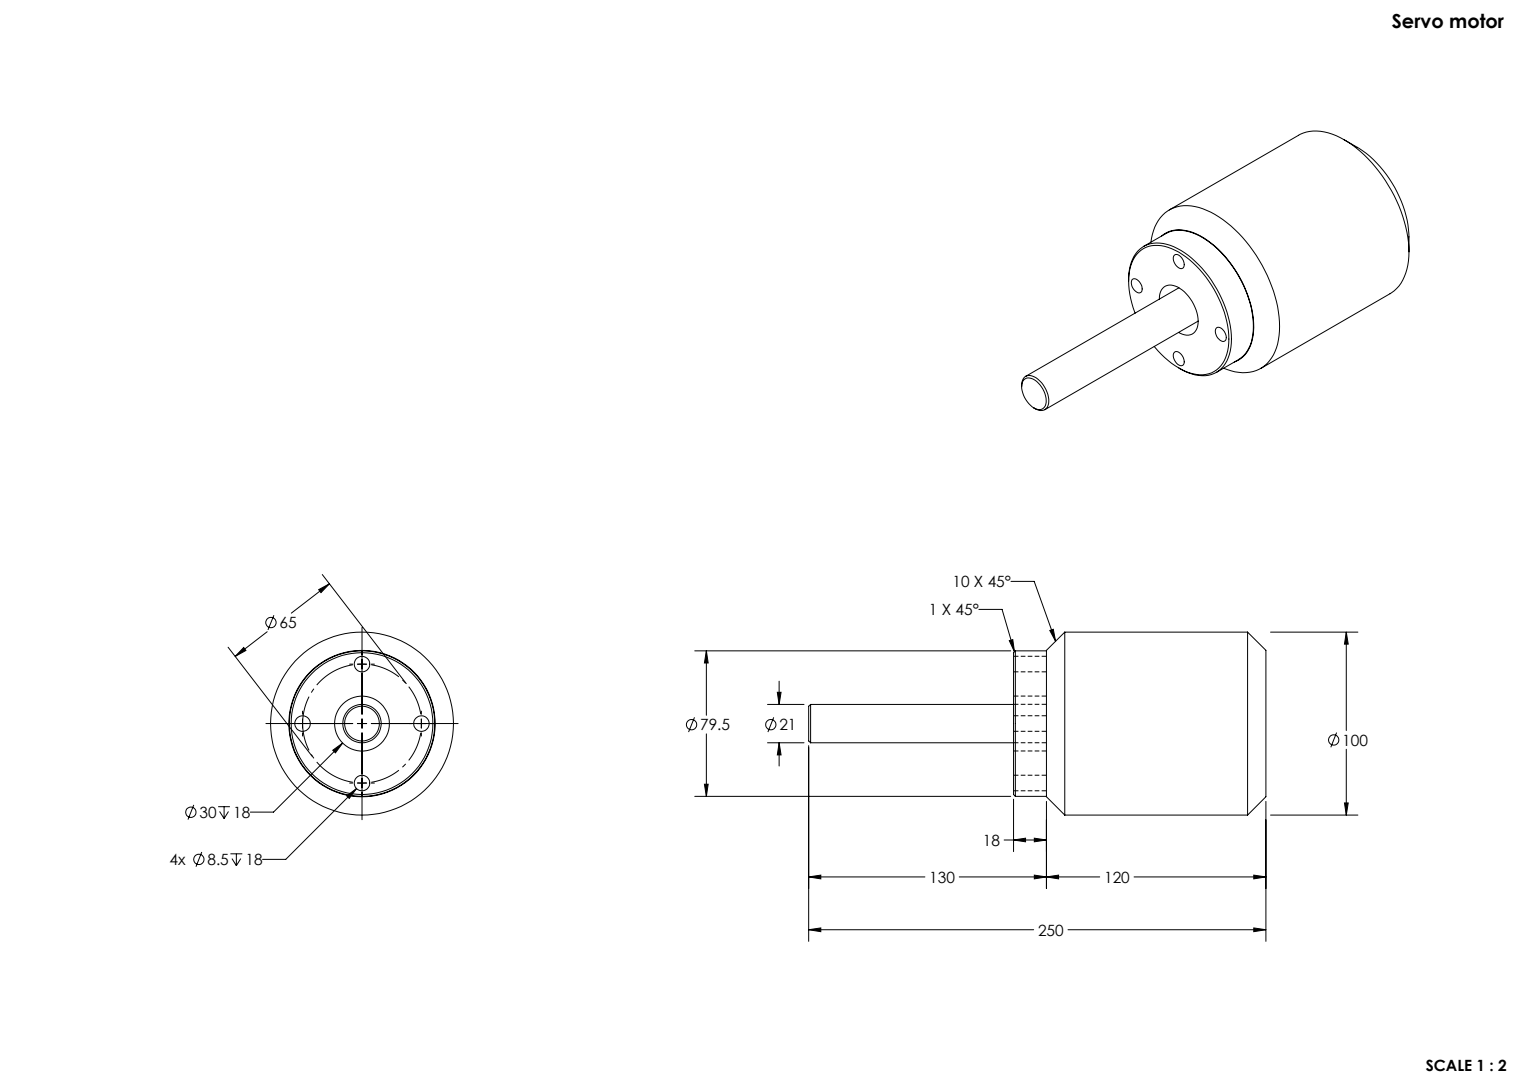
ISO-10303-21;
HEADER;
FILE_DESCRIPTION (('STEP AP214'),
    '1' );
FILE_NAME ('Servo motor.step',
    '2026-10-24T15:53:57',
    ( '' ),
    ( '' ),
    'SwSTEP 2.0',
    'SolidWorks 2025',
    '' );
FILE_SCHEMA (( 'AUTOMOTIVE_DESIGN' ));
ENDSEC;

DATA;
#2=DIRECTION ( 'NONE',  ( -3.851859888774471706E-33, -1.232595164407830946E-32, -1.000000000000000000 ) ) ;
#12=CONICAL_SURFACE ( 'NONE', #4068, 9.499999999999998224, 0.7853981633974257415 ) ;
#15=CIRCLE ( 'NONE', #7701, 10.50000000000002132 ) ;
#24=CARTESIAN_POINT ( 'NONE',  ( 28.24999999999996092, 1.387778780781445676E-14, 18.00000000000000355 ) ) ;
#39=EDGE_CURVE ( 'NONE', #7000, #2703, #3383, .T. ) ;
#42=ORIENTED_EDGE ( 'NONE', *, *, #2072, .T. ) ;
#43=CARTESIAN_POINT ( 'NONE',  ( 15.00000000000000000, 1.836970198721029589E-15, -4.814824860968080875E-32 ) ) ;
#49=DIRECTION ( 'NONE',  ( 3.851859888774471706E-33, -7.598173571352223877E-18, 1.000000000000000000 ) ) ;
#50=ORIENTED_EDGE ( 'NONE', *, *, #3725, .T. ) ;
#58=DIRECTION ( 'NONE',  ( -3.851859888774471706E-33, 7.598173571352223877E-18, -1.000000000000000000 ) ) ;
#68=ORIENTED_EDGE ( 'NONE', *, *, #5960, .T. ) ;
#70=CIRCLE ( 'NONE', #2861, 15.00000000000002487 ) ;
#72=DIRECTION ( 'NONE',  ( -3.851859888774471706E-33, 7.598173571352223877E-18, -1.000000000000000000 ) ) ;
#115=CIRCLE ( 'NONE', #6125, 4.250000000000013323 ) ;
#134=AXIS2_PLACEMENT_3D ( 'NONE', #4752, #7312, #2784 ) ;
#145=FACE_OUTER_BOUND ( 'NONE', #4016, .T. ) ;
#151=CARTESIAN_POINT ( 'NONE',  ( 39.75000000000007105, 4.867971026610737916E-15, 18.00000000000000355 ) ) ;
#169=DIRECTION ( 'NONE',  ( -3.851859888774471706E-33, -1.232595164407830946E-32, -1.000000000000000000 ) ) ;
#226=VECTOR ( 'NONE', #5474, 1000.000000000000000 ) ;
#227=DIRECTION ( 'NONE',  ( -3.851859888774471706E-33, 7.598173571352223877E-18, -1.000000000000000000 ) ) ;
#235=LINE ( 'NONE', #7430, #3287 ) ;
#241=DIRECTION ( 'NONE',  ( 3.851859888774471706E-33, -7.598173571352223877E-18, 1.000000000000000000 ) ) ;
#245=EDGE_CURVE ( 'NONE', #3380, #4181, #3653, .T. ) ;
#271=AXIS2_PLACEMENT_3D ( 'NONE', #6647, #2, #2074 ) ;
#278=CIRCLE ( 'NONE', #4737, 38.74999999999999289 ) ;
#279=AXIS2_PLACEMENT_3D ( 'NONE', #7241, #6496, #6681 ) ;
#283=DIRECTION ( 'NONE',  ( 1.000000000000000000, 0.000000000000000000, 0.000000000000000000 ) ) ;
#295=ORIENTED_EDGE ( 'NONE', *, *, #7376, .F. ) ;
#297=PRODUCT_DEFINITION ( 'UNKNOWN', '', #2849, #7006 ) ;
#311=EDGE_LOOP ( 'NONE', ( #3317, #6178 ) ) ;
#352=DIRECTION ( 'NONE',  ( -0.7071067811865456854, -8.706684567168461317E-33, -0.7071067811865493491 ) ) ;
#358=DIRECTION ( 'NONE',  ( -1.000000000000000000, 0.000000000000000000, 0.000000000000000000 ) ) ;
#364=DIRECTION ( 'NONE',  ( -6.400024471207001551E-36, 1.000000000000000000, 7.598173571352213092E-18 ) ) ;
#372=ADVANCED_FACE ( 'NONE', ( #5721 ), #1722, .F. ) ;
#394=EDGE_CURVE ( 'NONE', #7471, #7660, #2461, .T. ) ;
#397=DIRECTION ( 'NONE',  ( -3.851859888774471706E-33, -1.232595164407830946E-32, -1.000000000000000000 ) ) ;
#409=CARTESIAN_POINT ( 'NONE',  ( 2.560009788482798696E-34, -40.00000000000000711, -120.0000000000000000 ) ) ;
#412=AXIS2_PLACEMENT_3D ( 'NONE', #1063, #3836, #3059 ) ;
#416=CIRCLE ( 'NONE', #7358, 15.00000000000002487 ) ;
#422=ORIENTED_EDGE ( 'NONE', *, *, #2951, .T. ) ;
#425=VECTOR ( 'NONE', #4592, 1000.000000000000000 ) ;
#431=CIRCLE ( 'NONE', #5289, 4.250000000000010658 ) ;
#447=DIRECTION ( 'NONE',  ( 6.400024471207029615E-36, -1.000000000000000000, 0.000000000000000000 ) ) ;
#448=DIRECTION ( 'NONE',  ( -6.400024471207028278E-36, 1.000000000000000000, 0.000000000000000000 ) ) ;
#467=CARTESIAN_POINT ( 'NONE',  ( 1.163414459189985288E-15, -9.500000000000001776, 130.0000000000000000 ) ) ;
#468=AXIS2_PLACEMENT_3D ( 'NONE', #4578, #1260, #4007 ) ;
#473=CIRCLE ( 'NONE', #3101, 10.50000000000001066 ) ;
#474=ADVANCED_FACE ( 'NONE', ( #7871 ), #5260, .F. ) ;
#489=CARTESIAN_POINT ( 'NONE',  ( 0.000000000000000000, 0.000000000000000000, 18.00000000000000355 ) ) ;
#505=AXIS2_PLACEMENT_3D ( 'NONE', #1191, #6397, #7652 ) ;
#511=FACE_BOUND ( 'NONE', #2259, .T. ) ;
#518=PLANE ( 'NONE',  #4992 ) ;
#545=DIRECTION ( 'NONE',  ( 0.000000000000000000, -1.000000000000000000, -7.598173571352217714E-18 ) ) ;
#552=PRODUCT ( 'Servo motor', 'Servo motor', '', ( #3975 ) ) ;
#562=CARTESIAN_POINT ( 'NONE',  ( 0.000000000000000000, -32.50000000000004974, 0.000000000000000000 ) ) ;
#594=ORIENTED_EDGE ( 'NONE', *, *, #4710, .T. ) ;
#595=DIRECTION ( 'NONE',  ( -3.851859888774471706E-33, 7.598173571352223877E-18, -1.000000000000000000 ) ) ;
#607=ORIENTED_EDGE ( 'NONE', *, *, #3193, .T. ) ;
#623=EDGE_CURVE ( 'NONE', #2349, #7854, #2821, .T. ) ;
#634=CARTESIAN_POINT ( 'NONE',  ( 4.250000000000008882, -32.50000000000004974, 18.00000000000000355 ) ) ;
#651=CARTESIAN_POINT ( 'NONE',  ( -36.74999999999997158, 3.469446951953614189E-15, 18.00000000000000355 ) ) ;
#665=ADVANCED_FACE ( 'NONE', ( #7690 ), #1718, .F. ) ;
#667=CARTESIAN_POINT ( 'NONE',  ( -4.250000000000008882, -32.50000000000004974, 18.00000000000000355 ) ) ;
#679=CARTESIAN_POINT ( 'NONE',  ( -6.080023247646675662E-35, 9.499999999999994671, 130.0000000000000000 ) ) ;
#710=EDGE_CURVE ( 'NONE', #6028, #749, #1114, .T. ) ;
#721=DIRECTION ( 'NONE',  ( -3.851859888774471706E-33, -1.232595164407830946E-32, -1.000000000000000000 ) ) ;
#730=CONICAL_SURFACE ( 'NONE', #5761, 38.74999999999999289, 0.7853981633974447263 ) ;
#741=ORIENTED_EDGE ( 'NONE', *, *, #2143, .F. ) ;
#749=VERTEX_POINT ( 'NONE', #8210 ) ;
#775=DIRECTION ( 'NONE',  ( 6.400024471206997542E-36, -1.000000000000000000, -7.598173571352217714E-18 ) ) ;
#790=ORIENTED_EDGE ( 'NONE', *, *, #7457, .F. ) ;
#801=CIRCLE ( 'NONE', #5690, 50.00000000000008527 ) ;
#811=ORIENTED_EDGE ( 'NONE', *, *, #1222, .F. ) ;
#812=AXIS2_PLACEMENT_3D ( 'NONE', #2265, #397, #3583 ) ;
#823=PLANE ( 'NONE',  #3004 ) ;
#835=FACE_OUTER_BOUND ( 'NONE', #4264, .T. ) ;
#840=CONICAL_SURFACE ( 'NONE', #412, 40.00000000000007816, 0.7853981633974445042 ) ;
#869=DIRECTION ( 'NONE',  ( 3.851859888774471706E-33, -7.598173571352223877E-18, 1.000000000000000000 ) ) ;
#875=EDGE_CURVE ( 'NONE', #8340, #3886, #3801, .T. ) ;
#879=ORIENTED_EDGE ( 'NONE', *, *, #2756, .T. ) ;
#906=ORIENTED_EDGE ( 'NONE', *, *, #2537, .F. ) ;
#922=VERTEX_POINT ( 'NONE', #6767 ) ;
#923=ORIENTED_EDGE ( 'NONE', *, *, #1782, .F. ) ;
#939=CARTESIAN_POINT ( 'NONE',  ( 0.000000000000000000, -3.469446951953614189E-15, 130.0000000000000000 ) ) ;
#945=( LENGTH_UNIT ( ) NAMED_UNIT ( * ) SI_UNIT ( .MILLI., .METRE. ) );
#946=ORIENTED_EDGE ( 'NONE', *, *, #5359, .T. ) ;
#956=ORIENTED_EDGE ( 'NONE', *, *, #7414, .F. ) ;
#958=EDGE_LOOP ( 'NONE', ( #3855, #811 ) ) ;
#970=CARTESIAN_POINT ( 'NONE',  ( -28.24999999999997513, 3.989921841591238568E-15, 18.00000000000000355 ) ) ;
#979=AXIS2_PLACEMENT_3D ( 'NONE', #2979, #8205, #1025 ) ;
#981=AXIS2_PLACEMENT_3D ( 'NONE', #6340, #5095, #364 ) ;
#1003=LINE ( 'NONE', #6324, #6738 ) ;
#1005=PLANE ( 'NONE',  #2797 ) ;
#1014=ADVANCED_FACE ( 'NONE', ( #835 ), #3488, .F. ) ;
#1025=DIRECTION ( 'NONE',  ( 1.000000000000000000, 0.000000000000000000, 0.000000000000000000 ) ) ;
#1028=DIRECTION ( 'NONE',  ( 6.400024471207000214E-36, -1.000000000000000000, 0.000000000000000000 ) ) ;
#1029=ADVANCED_FACE ( 'NONE', ( #8280, #2872 ), #5541, .T. ) ;
#1038=EDGE_LOOP ( 'NONE', ( #6111, #1879 ) ) ;
#1052=AXIS2_PLACEMENT_3D ( 'NONE', #2524, #6525, #3174 ) ;
#1057=ADVANCED_FACE ( 'NONE', ( #6242 ), #5780, .T. ) ;
#1063=CARTESIAN_POINT ( 'NONE',  ( 0.000000000000000000, 0.000000000000000000, 0.000000000000000000 ) ) ;
#1067=LINE ( 'NONE', #4415, #4716 ) ;
#1085=DIRECTION ( 'NONE',  ( 6.400024471206996205E-36, -1.000000000000000000, -7.598173571352216173E-18 ) ) ;
#1114=LINE ( 'NONE', #467, #1443 ) ;
#1123=ORIENTED_EDGE ( 'NONE', *, *, #5960, .F. ) ;
#1143=ORIENTED_EDGE ( 'NONE', *, *, #1936, .T. ) ;
#1149=CARTESIAN_POINT ( 'NONE',  ( -15.00000000000002487, 1.926036882627243013E-34, 18.00000000000000355 ) ) ;
#1176=ORIENTED_EDGE ( 'NONE', *, *, #245, .T. ) ;
#1183=EDGE_LOOP ( 'NONE', ( #5544, #5968 ) ) ;
#1191=CARTESIAN_POINT ( 'NONE',  ( 0.000000000000000000, 0.000000000000000000, 0.000000000000000000 ) ) ;
#1199=AXIS2_PLACEMENT_3D ( 'NONE', #4817, #4940, #4156 ) ;
#1207=FACE_OUTER_BOUND ( 'NONE', #4849, .T. ) ;
#1222=EDGE_CURVE ( 'NONE', #7754, #1987, #70, .T. ) ;
#1226=EDGE_LOOP ( 'NONE', ( #2572, #6026, #2747, #6490 ) ) ;
#1233=VECTOR ( 'NONE', #2637, 999.9999999999998863 ) ;
#1248=ORIENTED_EDGE ( 'NONE', *, *, #1592, .T. ) ;
#1260=DIRECTION ( 'NONE',  ( 3.851859888774471706E-33, -7.598173571352223877E-18, 1.000000000000000000 ) ) ;
#1276=ADVANCED_FACE ( 'NONE', ( #3343 ), #2439, .T. ) ;
#1285=DIRECTION ( 'NONE',  ( 6.400024471206996205E-36, -1.000000000000000000, -7.598173571352216173E-18 ) ) ;
#1312=FACE_BOUND ( 'NONE', #1183, .T. ) ;
#1319=( LENGTH_UNIT ( ) NAMED_UNIT ( * ) SI_UNIT ( .MILLI., .METRE. ) );
#1322=ORIENTED_EDGE ( 'NONE', *, *, #3699, .F. ) ;
#1334=CARTESIAN_POINT ( 'NONE',  ( 0.000000000000000000, 0.000000000000000000, 16.99999999999991829 ) ) ;
#1349=ORIENTED_EDGE ( 'NONE', *, *, #8404, .T. ) ;
#1360=SHAPE_DEFINITION_REPRESENTATION ( #8544, #5506 ) ;
#1362=ADVANCED_FACE ( 'NONE', ( #4951 ), #823, .T. ) ;
#1367=ORIENTED_EDGE ( 'NONE', *, *, #3136, .T. ) ;
#1374=DIRECTION ( 'NONE',  ( 6.400024471206996205E-36, -1.000000000000000000, 0.000000000000000000 ) ) ;
#1376=ORIENTED_EDGE ( 'NONE', *, *, #1782, .T. ) ;
#1403=CARTESIAN_POINT ( 'NONE',  ( 0.000000000000000000, 0.000000000000000000, -109.9999999999999574 ) ) ;
#1443=VECTOR ( 'NONE', #3114, 999.9999999999998863 ) ;
#1486=MECHANICAL_DESIGN_GEOMETRIC_PRESENTATION_REPRESENTATION('',(#4405),#7100);
#1488=AXIS2_PLACEMENT_3D ( 'NONE', #3281, #1937, #5297 ) ;
#1492=CARTESIAN_POINT ( 'NONE',  ( 1.285879139104719647E-15, 10.49999999999998934, 128.9999999999999432 ) ) ;
#1500=ORIENTED_EDGE ( 'NONE', *, *, #2789, .T. ) ;
#1501=DIRECTION ( 'NONE',  ( -3.851859888774471706E-33, 7.598173571352219255E-18, -1.000000000000000000 ) ) ;
#1529=CIRCLE ( 'NONE', #134, 9.499999999999998224 ) ;
#1530=ORIENTED_EDGE ( 'NONE', *, *, #1704, .F. ) ;
#1542=DIRECTION ( 'NONE',  ( 1.000000000000000000, 0.000000000000000000, 0.000000000000000000 ) ) ;
#1555=ORIENTED_EDGE ( 'NONE', *, *, #5156, .T. ) ;
#1556=DIRECTION ( 'NONE',  ( 1.000000000000000000, 0.000000000000000000, 0.000000000000000000 ) ) ;
#1565=FACE_OUTER_BOUND ( 'NONE', #5122, .T. ) ;
#1575=DIRECTION ( 'NONE',  ( 3.851859888774471706E-33, -7.598173571352223877E-18, 1.000000000000000000 ) ) ;
#1591=ORIENTED_EDGE ( 'NONE', *, *, #4375, .F. ) ;
#1592=EDGE_CURVE ( 'NONE', #2559, #2703, #6913, .T. ) ;
#1599=CARTESIAN_POINT ( 'NONE',  ( 0.000000000000000000, 0.000000000000000000, 0.000000000000000000 ) ) ;
#1625=ORIENTED_EDGE ( 'NONE', *, *, #7457, .T. ) ;
#1645=FACE_OUTER_BOUND ( 'NONE', #6219, .T. ) ;
#1659=CYLINDRICAL_SURFACE ( 'NONE', #4214, 50.00000000000008527 ) ;
#1664=CARTESIAN_POINT ( 'NONE',  ( 38.74999999999992184, 4.806738686653357720E-15, 18.00000000000000355 ) ) ;
#1667=EDGE_LOOP ( 'NONE', ( #2472, #3550, #7880, #5878 ) ) ;
#1669=DIRECTION ( 'NONE',  ( -3.851859888774471706E-33, 7.598173571352223877E-18, -1.000000000000000000 ) ) ;
#1687=CIRCLE ( 'NONE', #4903, 39.99999999999999289 ) ;
#1696=FACE_OUTER_BOUND ( 'NONE', #1842, .T. ) ;
#1704=EDGE_CURVE ( 'NONE', #5825, #7684, #7052, .T. ) ;
#1707=AXIS2_PLACEMENT_3D ( 'NONE', #7537, #8149, #7494 ) ;
#1718=CYLINDRICAL_SURFACE ( 'NONE', #1848, 4.250000000000008882 ) ;
#1722=CYLINDRICAL_SURFACE ( 'NONE', #3508, 4.250000000000014211 ) ;
#1733=CARTESIAN_POINT ( 'NONE',  ( -32.49999999999997158, 3.469446951953614189E-15, -6.938893903907228378E-15 ) ) ;
#1751=ORIENTED_EDGE ( 'NONE', *, *, #2831, .T. ) ;
#1768=CYLINDRICAL_SURFACE ( 'NONE', #5918, 39.75000000000007105 ) ;
#1780=DIRECTION ( 'NONE',  ( -3.851859888774471706E-33, 7.598173571352185358E-18, -1.000000000000000000 ) ) ;
#1781=FACE_OUTER_BOUND ( 'NONE', #2379, .T. ) ;
#1782=EDGE_CURVE ( 'NONE', #7684, #7000, #6953, .T. ) ;
#1794=EDGE_CURVE ( 'NONE', #4055, #4496, #5386, .T. ) ;
#1798=CIRCLE ( 'NONE', #271, 39.75000000000007105 ) ;
#1799=AXIS2_PLACEMENT_3D ( 'NONE', #4331, #2355, #2887 ) ;
#1811=CIRCLE ( 'NONE', #6412, 4.250000000000010658 ) ;
#1816=ORIENTED_EDGE ( 'NONE', *, *, #8022, .T. ) ;
#1817=CARTESIAN_POINT ( 'NONE',  ( 0.000000000000000000, 0.000000000000000000, 0.000000000000000000 ) ) ;
#1836=CIRCLE ( 'NONE', #2402, 39.75000000000007105 ) ;
#1841=SHAPE_REPRESENTATION_RELATIONSHIP ( 'NONE' , 'NONE' ,  #5506, #5949 ) ;
#1842=EDGE_LOOP ( 'NONE', ( #2326, #7663, #956, #5195 ) ) ;
#1847=EDGE_CURVE ( 'NONE', #922, #4055, #235, .T. ) ;
#1848=AXIS2_PLACEMENT_3D ( 'NONE', #4387, #5672, #5803 ) ;
#1850=CARTESIAN_POINT ( 'NONE',  ( 32.49999999999997158, 1.387778780781445676E-14, 18.00000000000000355 ) ) ;
#1860=ADVANCED_FACE ( 'NONE', ( #145 ), #3158, .T. ) ;
#1866=ORIENTED_EDGE ( 'NONE', *, *, #6415, .F. ) ;
#1879=ORIENTED_EDGE ( 'NONE', *, *, #2820, .T. ) ;
#1886=AXIS2_PLACEMENT_3D ( 'NONE', #4613, #5940, #8007 ) ;
#1905=FACE_OUTER_BOUND ( 'NONE', #5900, .T. ) ;
#1907=CARTESIAN_POINT ( 'NONE',  ( -38.74999999999992184, -5.658996171085535125E-33, 18.00000000000000355 ) ) ;
#1917=DIRECTION ( 'NONE',  ( 3.851859888774471706E-33, -7.598173571352223877E-18, 1.000000000000000000 ) ) ;
#1924=DIRECTION ( 'NONE',  ( 3.851859888774471706E-33, 1.232595164407830946E-32, 1.000000000000000000 ) ) ;
#1933=ORIENTED_EDGE ( 'NONE', *, *, #7521, .T. ) ;
#1936=EDGE_CURVE ( 'NONE', #2349, #2603, #3753, .T. ) ;
#1937=DIRECTION ( 'NONE',  ( 3.851859888774471706E-33, 1.232595164407830946E-32, 1.000000000000000000 ) ) ;
#1939=DIRECTION ( 'NONE',  ( -3.851859888774471706E-33, 7.598173571352223877E-18, -1.000000000000000000 ) ) ;
#1945=CARTESIAN_POINT ( 'NONE',  ( 0.000000000000000000, 32.50000000000005684, -6.938893903907228378E-15 ) ) ;
#1953=ORIENTED_EDGE ( 'NONE', *, *, #875, .F. ) ;
#1963=FACE_BOUND ( 'NONE', #8536, .T. ) ;
#1975=AXIS2_PLACEMENT_3D ( 'NONE', #562, #72, #5946 ) ;
#1979=EDGE_CURVE ( 'NONE', #6357, #6260, #416, .T. ) ;
#1987=VERTEX_POINT ( 'NONE', #5663 ) ;
#2050=CARTESIAN_POINT ( 'NONE',  ( -2.560009788482805538E-34, 40.00000000000007816, 3.039269428540890907E-16 ) ) ;
#2056=( NAMED_UNIT ( * ) PLANE_ANGLE_UNIT ( ) SI_UNIT ( $, .RADIAN. ) );
#2057=DIRECTION ( 'NONE',  ( 1.000000000000000000, 0.000000000000000000, 0.000000000000000000 ) ) ;
#2062=EDGE_LOOP ( 'NONE', ( #3028, #7325 ) ) ;
#2072=EDGE_CURVE ( 'NONE', #8340, #7867, #1067, .T. ) ;
#2074=DIRECTION ( 'NONE',  ( 1.000000000000000000, -1.284024588418159550E-35, 0.000000000000000000 ) ) ;
#2085=CARTESIAN_POINT ( 'NONE',  ( 28.24999999999996803, 1.387778780781445676E-14, 1.504632769052525000E-32 ) ) ;
#2088=AXIS2_PLACEMENT_3D ( 'NONE', #3246, #58, #1285 ) ;
#2093=VERTEX_POINT ( 'NONE', #3767 ) ;
#2100=AXIS2_PLACEMENT_3D ( 'NONE', #6199, #5587, #1556 ) ;
#2109=ORIENTED_EDGE ( 'NONE', *, *, #1847, .F. ) ;
#2133=DIRECTION ( 'NONE',  ( 3.851859888774471706E-33, 1.232595164407830946E-32, 1.000000000000000000 ) ) ;
#2137=VECTOR ( 'NONE', #5924, 1000.000000000000000 ) ;
#2138=DIRECTION ( 'NONE',  ( 3.851859888774471706E-33, -7.598173571352216173E-18, 1.000000000000000000 ) ) ;
#2143=EDGE_CURVE ( 'NONE', #7867, #749, #8052, .T. ) ;
#2149=LINE ( 'NONE', #2050, #4965 ) ;
#2180=DIRECTION ( 'NONE',  ( -1.000000000000000000, 0.000000000000000000, 0.000000000000000000 ) ) ;
#2204=LINE ( 'NONE', #5565, #5002 ) ;
#2241=DIRECTION ( 'NONE',  ( 3.851859888774471706E-33, 1.232595164407830946E-32, 1.000000000000000000 ) ) ;
#2243=CARTESIAN_POINT ( 'NONE',  ( 0.000000000000000000, 0.000000000000000000, -10.00000000000006395 ) ) ;
#2259=EDGE_LOOP ( 'NONE', ( #8257, #2990 ) ) ;
#2265=CARTESIAN_POINT ( 'NONE',  ( -32.49999999999997158, 3.469446951953614189E-15, 18.00000000000000355 ) ) ;
#2271=AXIS2_PLACEMENT_3D ( 'NONE', #4493, #7984, #4632 ) ;
#2273=ADVANCED_FACE ( 'NONE', ( #1781 ), #3757, .F. ) ;
#2276=DIRECTION ( 'NONE',  ( -1.000000000000000000, 0.000000000000000000, 0.000000000000000000 ) ) ;
#2307=EDGE_LOOP ( 'NONE', ( #1322, #4419 ) ) ;
#2308=DIRECTION ( 'NONE',  ( -3.851859888774471706E-33, 7.598173571352185358E-18, -1.000000000000000000 ) ) ;
#2320=CARTESIAN_POINT ( 'NONE',  ( 0.000000000000000000, 0.000000000000000000, -109.9999999999999574 ) ) ;
#2326=ORIENTED_EDGE ( 'NONE', *, *, #4473, .F. ) ;
#2328=ORIENTED_EDGE ( 'NONE', *, *, #1794, .F. ) ;
#2335=FACE_OUTER_BOUND ( 'NONE', #3132, .T. ) ;
#2340=DIRECTION ( 'NONE',  ( 6.400024471206996205E-36, -1.000000000000000000, -7.598173571352216173E-18 ) ) ;
#2349=VERTEX_POINT ( 'NONE', #970 ) ;
#2354=VECTOR ( 'NONE', #2732, 1000.000000000000000 ) ;
#2355=DIRECTION ( 'NONE',  ( -3.851859888774471706E-33, 7.598173571352223877E-18, -1.000000000000000000 ) ) ;
#2379=EDGE_LOOP ( 'NONE', ( #1555, #6607 ) ) ;
#2380=DIRECTION ( 'NONE',  ( 6.400024471206996205E-36, -1.000000000000000000, -7.598173571352216173E-18 ) ) ;
#2383=AXIS2_PLACEMENT_3D ( 'NONE', #5965, #8595, #5207 ) ;
#2387=DIRECTION ( 'NONE',  ( 3.851859888774471706E-33, -7.598173571352216173E-18, 1.000000000000000000 ) ) ;
#2402=AXIS2_PLACEMENT_3D ( 'NONE', #4004, #4668, #7922 ) ;
#2410=CIRCLE ( 'NONE', #2972, 40.00000000000007816 ) ;
#2417=ORIENTED_EDGE ( 'NONE', *, *, #2820, .F. ) ;
#2434=EDGE_LOOP ( 'NONE', ( #2417, #1376, #8490, #6841 ) ) ;
#2436=DIRECTION ( 'NONE',  ( 6.400024471206993532E-36, -1.000000000000000000, -7.598173571352213092E-18 ) ) ;
#2439=CONICAL_SURFACE ( 'NONE', #1886, 50.00000000000008527, 0.7853981633974497223 ) ;
#2456=EDGE_LOOP ( 'NONE', ( #7051, #6209, #1816, #594 ) ) ;
#2461=LINE ( 'NONE', #5112, #7266 ) ;
#2472=ORIENTED_EDGE ( 'NONE', *, *, #1979, .T. ) ;
#2476=ORIENTED_EDGE ( 'NONE', *, *, #5969, .T. ) ;
#2491=CIRCLE ( 'NONE', #7361, 50.00000000000008527 ) ;
#2496=ADVANCED_FACE ( 'NONE', ( #3546 ), #6256, .F. ) ;
#2514=DIRECTION ( 'NONE',  ( -3.851859888774471706E-33, -1.232595164407830946E-32, -1.000000000000000000 ) ) ;
#2524=CARTESIAN_POINT ( 'NONE',  ( 0.000000000000000000, -3.469446951953614189E-15, 130.0000000000000000 ) ) ;
#2526=PLANE ( 'NONE',  #4830 ) ;
#2537=EDGE_CURVE ( 'NONE', #4358, #7854, #5861, .T. ) ;
#2559=VERTEX_POINT ( 'NONE', #6991 ) ;
#2572=ORIENTED_EDGE ( 'NONE', *, *, #7492, .F. ) ;
#2574=FACE_BOUND ( 'NONE', #2062, .T. ) ;
#2576=CARTESIAN_POINT ( 'NONE',  ( -15.00000000000000000, -1.107409611084418900E-31, 18.00000000000000355 ) ) ;
#2586=ORIENTED_EDGE ( 'NONE', *, *, #4901, .T. ) ;
#2587=ADVANCED_FACE ( 'NONE', ( #1696 ), #840, .T. ) ;
#2603=VERTEX_POINT ( 'NONE', #651 ) ;
#2630=VERTEX_POINT ( 'NONE', #4411 ) ;
#2631=CYLINDRICAL_SURFACE ( 'NONE', #4351, 10.50000000000001066 ) ;
#2637=DIRECTION ( 'NONE',  ( -2.728201748236299157E-33, 0.7071067811865321406, -0.7071067811865628938 ) ) ;
#2671=DIRECTION ( 'NONE',  ( -1.000000000000000000, 1.284024588418159550E-35, 0.000000000000000000 ) ) ;
#2677=AXIS2_PLACEMENT_3D ( 'NONE', #4713, #7529, #8177 ) ;
#2703=VERTEX_POINT ( 'NONE', #2828 ) ;
#2712=ORIENTED_EDGE ( 'NONE', *, *, #5928, .T. ) ;
#2732=DIRECTION ( 'NONE',  ( -3.851859888774471706E-33, -1.232595164407830946E-32, -1.000000000000000000 ) ) ;
#2734=CARTESIAN_POINT ( 'NONE',  ( 32.49999999999997158, 1.387778780781445676E-14, 0.000000000000000000 ) ) ;
#2740=AXIS2_PLACEMENT_3D ( 'NONE', #3295, #5307, #4041 ) ;
#2747=ORIENTED_EDGE ( 'NONE', *, *, #1847, .T. ) ;
#2756=EDGE_CURVE ( 'NONE', #7472, #6028, #1529, .T. ) ;
#2761=CARTESIAN_POINT ( 'NONE',  ( 0.000000000000000000, -3.469446951953614189E-15, 130.0000000000000000 ) ) ;
#2770=CARTESIAN_POINT ( 'NONE',  ( 0.000000000000000000, -3.469446951953614189E-15, 130.0000000000000000 ) ) ;
#2784=DIRECTION ( 'NONE',  ( 6.400024471206996205E-36, -1.000000000000000000, 0.000000000000000000 ) ) ;
#2789=EDGE_CURVE ( 'NONE', #5471, #3289, #7370, .T. ) ;
#2797=AXIS2_PLACEMENT_3D ( 'NONE', #8275, #3038, #2380 ) ;
#2799=CARTESIAN_POINT ( 'NONE',  ( 0.000000000000000000, 0.000000000000000000, 18.00000000000000355 ) ) ;
#2816=VERTEX_POINT ( 'NONE', #7015 ) ;
#2820=EDGE_CURVE ( 'NONE', #7684, #5825, #278, .T. ) ;
#2821=LINE ( 'NONE', #5486, #6047 ) ;
#2828=CARTESIAN_POINT ( 'NONE',  ( 39.75000000000000000, 4.867971026610730028E-15, 0.000000000000000000 ) ) ;
#2831=EDGE_CURVE ( 'NONE', #2603, #2349, #5871, .T. ) ;
#2845=ORIENTED_EDGE ( 'NONE', *, *, #4946, .T. ) ;
#2849=PRODUCT_DEFINITION_FORMATION_WITH_SPECIFIED_SOURCE ( 'ANY', '', #552, .NOT_KNOWN. ) ;
#2861=AXIS2_PLACEMENT_3D ( 'NONE', #1817, #7056, #1085 ) ;
#2872=FACE_OUTER_BOUND ( 'NONE', #958, .T. ) ;
#2879=ADVANCED_FACE ( 'NONE', ( #5538 ), #1005, .T. ) ;
#2884=DIRECTION ( 'NONE',  ( 0.000000000000000000, -1.000000000000000000, -7.598173571352319403E-18 ) ) ;
#2886=ORIENTED_EDGE ( 'NONE', *, *, #5180, .F. ) ;
#2887=DIRECTION ( 'NONE',  ( 6.400024471206997542E-36, -1.000000000000000000, 0.000000000000000000 ) ) ;
#2892=DIRECTION ( 'NONE',  ( -3.851859888774471706E-33, -1.232595164407830946E-32, -1.000000000000000000 ) ) ;
#2893=ORIENTED_EDGE ( 'NONE', *, *, #5359, .F. ) ;
#2894=DIRECTION ( 'NONE',  ( 3.851859888774471706E-33, 1.232595164407830946E-32, 1.000000000000000000 ) ) ;
#2908=AXIS2_PLACEMENT_3D ( 'NONE', #7026, #3716, #6298 ) ;
#2919=CIRCLE ( 'NONE', #1799, 39.99999999999999289 ) ;
#2935=CARTESIAN_POINT ( 'NONE',  ( 4.250000000000000888, 32.50000000000005684, 18.00000000000000355 ) ) ;
#2948=CARTESIAN_POINT ( 'NONE',  ( 0.000000000000000000, 0.000000000000000000, 0.000000000000000000 ) ) ;
#2951=EDGE_CURVE ( 'NONE', #4496, #4055, #1811, .T. ) ;
#2956=CIRCLE ( 'NONE', #1975, 4.250000000000010658 ) ;
#2972=AXIS2_PLACEMENT_3D ( 'NONE', #1599, #869, #2997 ) ;
#2979=CARTESIAN_POINT ( 'NONE',  ( 0.000000000000000000, 32.50000000000005684, 18.00000000000000355 ) ) ;
#2990=ORIENTED_EDGE ( 'NONE', *, *, #4325, .F. ) ;
#2997=DIRECTION ( 'NONE',  ( 6.400024471206997542E-36, -1.000000000000000000, -7.598173571352216173E-18 ) ) ;
#3004=AXIS2_PLACEMENT_3D ( 'NONE', #2948, #2138, #6797 ) ;
#3007=CARTESIAN_POINT ( 'NONE',  ( 0.000000000000000000, -32.50000000000004974, 18.00000000000000355 ) ) ;
#3028=ORIENTED_EDGE ( 'NONE', *, *, #1979, .F. ) ;
#3031=EDGE_CURVE ( 'NONE', #6260, #6357, #3633, .T. ) ;
#3038=DIRECTION ( 'NONE',  ( 3.851859888774471706E-33, -7.598173571352216173E-18, 1.000000000000000000 ) ) ;
#3049=ADVANCED_FACE ( 'NONE', ( #4859 ), #730, .T. ) ;
#3051=UNCERTAINTY_MEASURE_WITH_UNIT (LENGTH_MEASURE( 1.000000000000000082E-05 ), #945, 'distance_accuracy_value', 'NONE');
#3059=DIRECTION ( 'NONE',  ( -6.400024471207001551E-36, 1.000000000000000000, 7.598173571352213092E-18 ) ) ;
#3064=DIRECTION ( 'NONE',  ( 3.851859888774471706E-33, 1.232595164407830946E-32, 1.000000000000000000 ) ) ;
#3072=LINE ( 'NONE', #7080, #4481 ) ;
#3082=ORIENTED_EDGE ( 'NONE', *, *, #8370, .F. ) ;
#3084=PLANE ( 'NONE',  #4433 ) ;
#3101=AXIS2_PLACEMENT_3D ( 'NONE', #5695, #2308, #447 ) ;
#3102=AXIS2_PLACEMENT_3D ( 'NONE', #5160, #7818, #5891 ) ;
#3114=DIRECTION ( 'NONE',  ( 8.659560562354746736E-17, -0.7071067811865321406, -0.7071067811865628938 ) ) ;
#3132=EDGE_LOOP ( 'NONE', ( #6247, #4922, #607, #7004 ) ) ;
#3134=DIRECTION ( 'NONE',  ( 0.000000000000000000, -1.000000000000000000, -7.598173571352319403E-18 ) ) ;
#3136=EDGE_CURVE ( 'NONE', #2816, #5332, #2956, .T. ) ;
#3158=CONICAL_SURFACE ( 'NONE', #7067, 9.499999999999998224, 0.7853981633974257415 ) ;
#3166=ORIENTED_EDGE ( 'NONE', *, *, #1936, .F. ) ;
#3174=DIRECTION ( 'NONE',  ( 6.400024471206997542E-36, -1.000000000000000000, 0.000000000000000000 ) ) ;
#3193=EDGE_CURVE ( 'NONE', #4094, #5811, #3304, .T. ) ;
#3222=FACE_BOUND ( 'NONE', #6447, .T. ) ;
#3226=ORIENTED_EDGE ( 'NONE', *, *, #623, .T. ) ;
#3241=AXIS2_PLACEMENT_3D ( 'NONE', #6891, #8318, #2340 ) ;
#3246=CARTESIAN_POINT ( 'NONE',  ( 0.000000000000000000, 0.000000000000000000, 0.000000000000000000 ) ) ;
#3252=ORIENTED_EDGE ( 'NONE', *, *, #3763, .T. ) ;
#3265=DIRECTION ( 'NONE',  ( 1.000000000000000000, -1.284024588418159550E-35, 3.851859888774464864E-33 ) ) ;
#3281=CARTESIAN_POINT ( 'NONE',  ( 0.000000000000000000, 0.000000000000000000, 18.00000000000000355 ) ) ;
#3287=VECTOR ( 'NONE', #2892, 1000.000000000000000 ) ;
#3289=VERTEX_POINT ( 'NONE', #6805 ) ;
#3295=CARTESIAN_POINT ( 'NONE',  ( 0.000000000000000000, 0.000000000000000000, 0.000000000000000000 ) ) ;
#3304=LINE ( 'NONE', #24, #7814 ) ;
#3315=CYLINDRICAL_SURFACE ( 'NONE', #4133, 39.75000000000007105 ) ;
#3317=ORIENTED_EDGE ( 'NONE', *, *, #8370, .T. ) ;
#3325=AXIS2_PLACEMENT_3D ( 'NONE', #4241, #227, #2884 ) ;
#3343=FACE_OUTER_BOUND ( 'NONE', #3806, .T. ) ;
#3364=EDGE_LOOP ( 'NONE', ( #2845, #7746, #8182, #1866 ) ) ;
#3380=VERTEX_POINT ( 'NONE', #5799 ) ;
#3383=LINE ( 'NONE', #151, #7105 ) ;
#3401=EDGE_CURVE ( 'NONE', #6357, #1987, #5106, .T. ) ;
#3444=EDGE_LOOP ( 'NONE', ( #4635, #1953 ) ) ;
#3450=EDGE_LOOP ( 'NONE', ( #7509, #5011, #8124, #6187 ) ) ;
#3451=LINE ( 'NONE', #5321, #7277 ) ;
#3484=ADVANCED_FACE ( 'NONE', ( #3845 ), #2631, .T. ) ;
#3488=CYLINDRICAL_SURFACE ( 'NONE', #7567, 4.250000000000003553 ) ;
#3495=FACE_OUTER_BOUND ( 'NONE', #4760, .T. ) ;
#3503=ORIENTED_EDGE ( 'NONE', *, *, #623, .F. ) ;
#3508=AXIS2_PLACEMENT_3D ( 'NONE', #1850, #4391, #3778 ) ;
#3512=DIRECTION ( 'NONE',  ( 1.000000000000000000, 0.000000000000000000, 0.000000000000000000 ) ) ;
#3523=ORIENTED_EDGE ( 'NONE', *, *, #4224, .F. ) ;
#3524=DIRECTION ( 'NONE',  ( 1.000000000000000000, 0.000000000000000000, 0.000000000000000000 ) ) ;
#3536=ORIENTED_EDGE ( 'NONE', *, *, #39, .F. ) ;
#3539=ADVANCED_FACE ( 'NONE', ( #4644 ), #7293, .F. ) ;
#3546=FACE_OUTER_BOUND ( 'NONE', #7900, .T. ) ;
#3550=ORIENTED_EDGE ( 'NONE', *, *, #6005, .T. ) ;
#3552=ORIENTED_EDGE ( 'NONE', *, *, #3929, .T. ) ;
#3560=EDGE_LOOP ( 'NONE', ( #2328, #7849 ) ) ;
#3564=CARTESIAN_POINT ( 'NONE',  ( 0.000000000000000000, 0.000000000000000000, 0.000000000000000000 ) ) ;
#3572=VERTEX_POINT ( 'NONE', #8036 ) ;
#3583=DIRECTION ( 'NONE',  ( -1.000000000000000000, 0.000000000000000000, 0.000000000000000000 ) ) ;
#3627=AXIS2_PLACEMENT_3D ( 'NONE', #6760, #6112, #3524 ) ;
#3628=CIRCLE ( 'NONE', #8346, 9.499999999999998224 ) ;
#3633=CIRCLE ( 'NONE', #4744, 15.00000000000002487 ) ;
#3642=ORIENTED_EDGE ( 'NONE', *, *, #39, .T. ) ;
#3646=VERTEX_POINT ( 'NONE', #3835 ) ;
#3653=CIRCLE ( 'NONE', #2677, 50.00000000000008527 ) ;
#3665=DIRECTION ( 'NONE',  ( -1.000000000000000000, 0.000000000000000000, 0.000000000000000000 ) ) ;
#3674=EDGE_LOOP ( 'NONE', ( #4253, #4809, #3552, #5634 ) ) ;
#3699=EDGE_CURVE ( 'NONE', #4094, #2093, #8382, .T. ) ;
#3710=FACE_OUTER_BOUND ( 'NONE', #5944, .T. ) ;
#3716=DIRECTION ( 'NONE',  ( 3.851859888774471706E-33, -7.598173571352216173E-18, 1.000000000000000000 ) ) ;
#3725=EDGE_CURVE ( 'NONE', #2603, #4358, #7282, .T. ) ;
#3740=DIRECTION ( 'NONE',  ( -1.000000000000000000, 1.284024588418159550E-35, 0.000000000000000000 ) ) ;
#3743=DIRECTION ( 'NONE',  ( 6.400024471206993532E-36, -1.000000000000000000, -7.598173571352311699E-18 ) ) ;
#3750=CARTESIAN_POINT ( 'NONE',  ( 4.250000000000000888, -32.50000000000004974, -1.504632769052525000E-32 ) ) ;
#3753=CIRCLE ( 'NONE', #5420, 4.250000000000007105 ) ;
#3757=PLANE ( 'NONE',  #2908 ) ;
#3763=EDGE_CURVE ( 'NONE', #3886, #8340, #15, .T. ) ;
#3764=CARTESIAN_POINT ( 'NONE',  ( 0.000000000000000000, -3.469446951953614189E-15, 130.0000000000000000 ) ) ;
#3767=CARTESIAN_POINT ( 'NONE',  ( 36.74999999999997868, 1.439826269745208429E-14, 18.00000000000000355 ) ) ;
#3778=DIRECTION ( 'NONE',  ( -1.000000000000000000, 0.000000000000000000, 0.000000000000000000 ) ) ;
#3801=CIRCLE ( 'NONE', #468, 10.50000000000002132 ) ;
#3803=DIRECTION ( 'NONE',  ( 1.000000000000000000, -1.284024588418159817E-35, 0.000000000000000000 ) ) ;
#3804=ORIENTED_EDGE ( 'NONE', *, *, #394, .F. ) ;
#3806=EDGE_LOOP ( 'NONE', ( #4930, #1933, #7641, #8233 ) ) ;
#3835=CARTESIAN_POINT ( 'NONE',  ( 36.74999999999997868, 1.439826269745208429E-14, -1.203706215242020903E-32 ) ) ;
#3836=DIRECTION ( 'NONE',  ( -3.851859888774471706E-33, 7.598173571352219255E-18, -1.000000000000000000 ) ) ;
#3845=FACE_OUTER_BOUND ( 'NONE', #6903, .T. ) ;
#3855=ORIENTED_EDGE ( 'NONE', *, *, #7344, .F. ) ;
#3879=EDGE_CURVE ( 'NONE', #7819, #4220, #1687, .T. ) ;
#3886=VERTEX_POINT ( 'NONE', #7005 ) ;
#3929=EDGE_CURVE ( 'NONE', #4220, #4181, #3072, .T. ) ;
#3955=DIRECTION ( 'NONE',  ( -3.851859888774471706E-33, -1.232595164407830946E-32, -1.000000000000000000 ) ) ;
#3972=ORIENTED_EDGE ( 'NONE', *, *, #710, .T. ) ;
#3975=PRODUCT_CONTEXT ( 'NONE', #5661, 'mechanical' ) ;
#3988=DIRECTION ( 'NONE',  ( 1.000000000000000000, -1.284024588418159550E-35, 0.000000000000000000 ) ) ;
#4004=CARTESIAN_POINT ( 'NONE',  ( 0.000000000000000000, 0.000000000000000000, 0.000000000000000000 ) ) ;
#4006=FACE_BOUND ( 'NONE', #2307, .T. ) ;
#4007=DIRECTION ( 'NONE',  ( 6.400024471206997542E-36, -1.000000000000000000, -7.598173571352217714E-18 ) ) ;
#4016=EDGE_LOOP ( 'NONE', ( #5883, #3972, #741, #4943 ) ) ;
#4029=LINE ( 'NONE', #634, #2354 ) ;
#4034=VECTOR ( 'NONE', #4767, 1000.000000000000000 ) ;
#4041=DIRECTION ( 'NONE',  ( 6.400024471206996205E-36, -1.000000000000000000, -7.598173571352216173E-18 ) ) ;
#4055=VERTEX_POINT ( 'NONE', #8593 ) ;
#4068=AXIS2_PLACEMENT_3D ( 'NONE', #5823, #1780, #448 ) ;
#4075=ORIENTED_EDGE ( 'NONE', *, *, #7376, .T. ) ;
#4094=VERTEX_POINT ( 'NONE', #8038 ) ;
#4133=AXIS2_PLACEMENT_3D ( 'NONE', #2799, #4630, #2671 ) ;
#4139=DIRECTION ( 'NONE',  ( 3.851859888774471706E-33, -7.598173571352220795E-18, 1.000000000000000000 ) ) ;
#4156=DIRECTION ( 'NONE',  ( 6.400024471206993532E-36, -1.000000000000000000, -7.598173571352311699E-18 ) ) ;
#4164=AXIS2_PLACEMENT_3D ( 'NONE', #7422, #6901, #2276 ) ;
#4181=VERTEX_POINT ( 'NONE', #7514 ) ;
#4203=CARTESIAN_POINT ( 'NONE',  ( 0.000000000000000000, 0.000000000000000000, 0.000000000000000000 ) ) ;
#4214=AXIS2_PLACEMENT_3D ( 'NONE', #3764, #1917, #4574 ) ;
#4220=VERTEX_POINT ( 'NONE', #409 ) ;
#4224=EDGE_CURVE ( 'NONE', #7660, #3572, #6866, .T. ) ;
#4232=VERTEX_POINT ( 'NONE', #2935 ) ;
#4241=CARTESIAN_POINT ( 'NONE',  ( -32.49999999999997158, 3.469446951953614189E-15, -6.938893903907228378E-15 ) ) ;
#4253=ORIENTED_EDGE ( 'NONE', *, *, #7521, .F. ) ;
#4255=ADVANCED_FACE ( 'NONE', ( #4372 ), #1659, .T. ) ;
#4261=CARTESIAN_POINT ( 'NONE',  ( 1.285879139104721028E-15, 10.50000000000000178, 7.978082249919836843E-17 ) ) ;
#4264=EDGE_LOOP ( 'NONE', ( #3503, #1143, #50, #8217 ) ) ;
#4269=CARTESIAN_POINT ( 'NONE',  ( -38.74999999999999289, 4.975595280120367735E-34, 18.00000000000000355 ) ) ;
#4286=DIRECTION ( 'NONE',  ( -3.851859888774471706E-33, 7.598173571352185358E-18, -1.000000000000000000 ) ) ;
#4291=( NAMED_UNIT ( * ) SI_UNIT ( $, .STERADIAN. ) SOLID_ANGLE_UNIT ( ) );
#4303=CARTESIAN_POINT ( 'NONE',  ( 39.75000000000000000, 4.867971026610730028E-15, 16.99999999999991829 ) ) ;
#4304=ADVANCED_FACE ( 'NONE', ( #8295 ), #5041, .T. ) ;
#4310=CIRCLE ( 'NONE', #5128, 4.250000000000013323 ) ;
#4313=DIRECTION ( 'NONE',  ( -1.000000000000000000, 0.000000000000000000, 0.000000000000000000 ) ) ;
#4321=CYLINDRICAL_SURFACE ( 'NONE', #4917, 4.250000000000008882 ) ;
#4325=EDGE_CURVE ( 'NONE', #2703, #2559, #1836, .T. ) ;
#4331=CARTESIAN_POINT ( 'NONE',  ( 0.000000000000000000, -1.040834085586084257E-14, -120.0000000000000000 ) ) ;
#4333=DIRECTION ( 'NONE',  ( 3.851859888774471706E-33, -7.598173571352220795E-18, 1.000000000000000000 ) ) ;
#4351=AXIS2_PLACEMENT_3D ( 'NONE', #2761, #49, #5337 ) ;
#4356=ORIENTED_EDGE ( 'NONE', *, *, #3136, .F. ) ;
#4358=VERTEX_POINT ( 'NONE', #8571 ) ;
#4372=FACE_OUTER_BOUND ( 'NONE', #3364, .T. ) ;
#4375=EDGE_CURVE ( 'NONE', #3380, #3572, #4796, .T. ) ;
#4387=CARTESIAN_POINT ( 'NONE',  ( 0.000000000000000000, 32.50000000000005684, 18.00000000000000355 ) ) ;
#4391=DIRECTION ( 'NONE',  ( -3.851859888774471706E-33, -1.232595164407830946E-32, -1.000000000000000000 ) ) ;
#4405=STYLED_ITEM('',(#8649),#5730);
#4411=CARTESIAN_POINT ( 'NONE',  ( -39.75000000000000000, -1.165861408448480429E-31, 16.99999999999991829 ) ) ;
#4415=CARTESIAN_POINT ( 'NONE',  ( 1.285879139104722211E-15, 10.50000000000000711, 130.0000000000000000 ) ) ;
#4419=ORIENTED_EDGE ( 'NONE', *, *, #8048, .F. ) ;
#4433=AXIS2_PLACEMENT_3D ( 'NONE', #5084, #5773, #7099 ) ;
#4473=EDGE_CURVE ( 'NONE', #7471, #4915, #5339, .T. ) ;
#4481=VECTOR ( 'NONE', #5757, 1000.000000000000227 ) ;
#4493=CARTESIAN_POINT ( 'NONE',  ( 0.000000000000000000, 0.000000000000000000, 0.000000000000000000 ) ) ;
#4496=VERTEX_POINT ( 'NONE', #7894 ) ;
#4514=ORIENTED_EDGE ( 'NONE', *, *, #7719, .F. ) ;
#4521=CIRCLE ( 'NONE', #8421, 4.250000000000010658 ) ;
#4527=CARTESIAN_POINT ( 'NONE',  ( 0.000000000000000000, -32.50000000000004974, 0.000000000000000000 ) ) ;
#4528=EDGE_CURVE ( 'NONE', #3289, #5471, #6188, .T. ) ;
#4547=EDGE_LOOP ( 'NONE', ( #923, #1530, #5754, #5422 ) ) ;
#4556=DIRECTION ( 'NONE',  ( -3.851859888774471706E-33, -1.232595164407830946E-32, -1.000000000000000000 ) ) ;
#4562=CARTESIAN_POINT ( 'NONE',  ( 0.000000000000000000, 0.000000000000000000, 18.00000000000000355 ) ) ;
#4567=AXIS2_PLACEMENT_3D ( 'NONE', #6332, #5688, #4313 ) ;
#4574=DIRECTION ( 'NONE',  ( 6.400024471206997542E-36, -1.000000000000000000, 0.000000000000000000 ) ) ;
#4578=CARTESIAN_POINT ( 'NONE',  ( 0.000000000000000000, 0.000000000000000000, 0.000000000000000000 ) ) ;
#4583=DIRECTION ( 'NONE',  ( 1.000000000000000000, 0.000000000000000000, 0.000000000000000000 ) ) ;
#4592=DIRECTION ( 'NONE',  ( -3.851859888774471706E-33, -1.232595164407830946E-32, -1.000000000000000000 ) ) ;
#4602=FACE_OUTER_BOUND ( 'NONE', #4839, .T. ) ;
#4613=CARTESIAN_POINT ( 'NONE',  ( 0.000000000000000000, 0.000000000000000000, -109.9999999999999574 ) ) ;
#4630=DIRECTION ( 'NONE',  ( -3.851859888774471706E-33, -1.232595164407830946E-32, -1.000000000000000000 ) ) ;
#4631=AXIS2_PLACEMENT_3D ( 'NONE', #5954, #1924, #4583 ) ;
#4632=DIRECTION ( 'NONE',  ( 6.400024471206997542E-36, -1.000000000000000000, -7.598173571352216173E-18 ) ) ;
#4633=AXIS2_PLACEMENT_3D ( 'NONE', #5792, #5228, #4976 ) ;
#4635=ORIENTED_EDGE ( 'NONE', *, *, #3763, .F. ) ;
#4637=CARTESIAN_POINT ( 'NONE',  ( 5.510910596163084034E-15, 39.99999999999992184, -120.0000000000000000 ) ) ;
#4644=FACE_OUTER_BOUND ( 'NONE', #3450, .T. ) ;
#4649=LINE ( 'NONE', #6692, #8503 ) ;
#4668=DIRECTION ( 'NONE',  ( 3.851859888774471706E-33, 1.232595164407830946E-32, 1.000000000000000000 ) ) ;
#4710=EDGE_CURVE ( 'NONE', #749, #7867, #473, .T. ) ;
#4713=CARTESIAN_POINT ( 'NONE',  ( 0.000000000000000000, 0.000000000000000000, -109.9999999999999574 ) ) ;
#4716=VECTOR ( 'NONE', #6999, 1000.000000000000000 ) ;
#4736=ORIENTED_EDGE ( 'NONE', *, *, #5380, .F. ) ;
#4737=AXIS2_PLACEMENT_3D ( 'NONE', #6368, #8232, #7053 ) ;
#4741=ADVANCED_FACE ( 'NONE', ( #1645 ), #4321, .F. ) ;
#4744=AXIS2_PLACEMENT_3D ( 'NONE', #5441, #2133, #8601 ) ;
#4752=CARTESIAN_POINT ( 'NONE',  ( 0.000000000000000000, -3.469446951953614189E-15, 130.0000000000000000 ) ) ;
#4760=EDGE_LOOP ( 'NONE', ( #2476, #3642, #7942, #7315 ) ) ;
#4767=DIRECTION ( 'NONE',  ( -3.851859888774471706E-33, -1.232595164407830946E-32, -1.000000000000000000 ) ) ;
#4779=DIRECTION ( 'NONE',  ( -3.851859888774471706E-33, -1.232595164407830946E-32, -1.000000000000000000 ) ) ;
#4796=LINE ( 'NONE', #5455, #6050 ) ;
#4802=ADVANCED_FACE ( 'NONE', ( #8573, #2574, #3222, #1312, #4006, #1963 ), #2526, .T. ) ;
#4809=ORIENTED_EDGE ( 'NONE', *, *, #5156, .F. ) ;
#4814=ORIENTED_EDGE ( 'NONE', *, *, #4224, .T. ) ;
#4817=CARTESIAN_POINT ( 'NONE',  ( 0.000000000000000000, 32.50000000000005684, -6.938893903907228378E-15 ) ) ;
#4819=LINE ( 'NONE', #8088, #6275 ) ;
#4830=AXIS2_PLACEMENT_3D ( 'NONE', #489, #5129, #3265 ) ;
#4839=EDGE_LOOP ( 'NONE', ( #1591, #1176, #7706, #4814 ) ) ;
#4849=EDGE_LOOP ( 'NONE', ( #879, #6759 ) ) ;
#4859=FACE_OUTER_BOUND ( 'NONE', #2434, .T. ) ;
#4872=DIRECTION ( 'NONE',  ( -3.851859888774471706E-33, -1.232595164407830946E-32, -1.000000000000000000 ) ) ;
#4874=CLOSED_SHELL ( 'NONE', ( #2587, #1276, #3049, #1860, #4255, #5728, #474, #6602, #6656, #372, #2496, #3484, #1029, #5317, #6785, #665, #8378, #4741, #1014, #3539, #8424, #4802, #5674, #2879, #1362, #6802, #2273, #6033, #8519, #6254, #1057, #4304, #8084 ) ) ;
#4879=CARTESIAN_POINT ( 'NONE',  ( -32.49999999999997158, 3.469446951953614189E-15, 18.00000000000000355 ) ) ;
#4887=CARTESIAN_POINT ( 'NONE',  ( 6.720025694767354167E-35, -10.50000000000001421, 130.0000000000000000 ) ) ;
#4899=DIRECTION ( 'NONE',  ( 6.400024471207000214E-36, -1.000000000000000000, 0.000000000000000000 ) ) ;
#4901=EDGE_CURVE ( 'NONE', #4915, #3572, #2149, .T. ) ;
#4903=AXIS2_PLACEMENT_3D ( 'NONE', #5670, #1669, #7607 ) ;
#4915=VERTEX_POINT ( 'NONE', #5499 ) ;
#4917=AXIS2_PLACEMENT_3D ( 'NONE', #3007, #6335, #358 ) ;
#4922=ORIENTED_EDGE ( 'NONE', *, *, #8048, .T. ) ;
#4930=ORIENTED_EDGE ( 'NONE', *, *, #3879, .F. ) ;
#4940=DIRECTION ( 'NONE',  ( -3.851859888774471706E-33, 7.598173571352223877E-18, -1.000000000000000000 ) ) ;
#4943=ORIENTED_EDGE ( 'NONE', *, *, #5928, .F. ) ;
#4946=EDGE_CURVE ( 'NONE', #4181, #3380, #801, .T. ) ;
#4951=FACE_OUTER_BOUND ( 'NONE', #7721, .T. ) ;
#4962=LINE ( 'NONE', #4269, #5546 ) ;
#4965=VECTOR ( 'NONE', #8109, 1000.000000000000227 ) ;
#4976=DIRECTION ( 'NONE',  ( 6.400024471207000214E-36, -1.000000000000000000, 0.000000000000000000 ) ) ;
#4992=AXIS2_PLACEMENT_3D ( 'NONE', #5173, #2387, #5121 ) ;
#5002=VECTOR ( 'NONE', #4779, 1000.000000000000000 ) ;
#5011=ORIENTED_EDGE ( 'NONE', *, *, #3031, .T. ) ;
#5035=CARTESIAN_POINT ( 'NONE',  ( 32.49999999999997158, 1.387778780781445676E-14, 0.000000000000000000 ) ) ;
#5041=CONICAL_SURFACE ( 'NONE', #6721, 50.00000000000008527, 0.7853981633974497223 ) ;
#5084=CARTESIAN_POINT ( 'NONE',  ( 0.000000000000000000, 0.000000000000000000, 0.000000000000000000 ) ) ;
#5095=DIRECTION ( 'NONE',  ( -3.851859888774471706E-33, 7.598173571352219255E-18, -1.000000000000000000 ) ) ;
#5106=LINE ( 'NONE', #1149, #2137 ) ;
#5112=CARTESIAN_POINT ( 'NONE',  ( 4.898587196589422492E-15, -40.00000000000007816, -3.039269428540890907E-16 ) ) ;
#5121=DIRECTION ( 'NONE',  ( 6.400024471206996205E-36, -1.000000000000000000, -7.598173571352216173E-18 ) ) ;
#5122=EDGE_LOOP ( 'NONE', ( #1751, #3226, #7039, #6783 ) ) ;
#5128=AXIS2_PLACEMENT_3D ( 'NONE', #2734, #1939, #7252 ) ;
#5129=DIRECTION ( 'NONE',  ( -3.851859888774464864E-33, 1.232595164407830946E-32, 1.000000000000000000 ) ) ;
#5156=EDGE_CURVE ( 'NONE', #4220, #7819, #2919, .T. ) ;
#5160=CARTESIAN_POINT ( 'NONE',  ( 0.000000000000000000, 0.000000000000000000, 0.000000000000000000 ) ) ;
#5173=CARTESIAN_POINT ( 'NONE',  ( 0.000000000000000000, 0.000000000000000000, 130.0000000000000000 ) ) ;
#5180=EDGE_CURVE ( 'NONE', #4232, #922, #7512, .T. ) ;
#5195=ORIENTED_EDGE ( 'NONE', *, *, #4901, .F. ) ;
#5207=DIRECTION ( 'NONE',  ( 6.400024471206997542E-36, -1.000000000000000000, 0.000000000000000000 ) ) ;
#5228=DIRECTION ( 'NONE',  ( -3.851859888774471706E-33, 7.598173571352219255E-18, -1.000000000000000000 ) ) ;
#5250=LINE ( 'NONE', #679, #1233 ) ;
#5260=CYLINDRICAL_SURFACE ( 'NONE', #5693, 15.00000000000002487 ) ;
#5289=AXIS2_PLACEMENT_3D ( 'NONE', #7676, #6990, #6457 ) ;
#5292=ORIENTED_EDGE ( 'NONE', *, *, #4528, .T. ) ;
#5297=DIRECTION ( 'NONE',  ( 1.000000000000000000, -1.284024588418159550E-35, 0.000000000000000000 ) ) ;
#5307=DIRECTION ( 'NONE',  ( 3.851859888774471706E-33, -7.598173571352216173E-18, 1.000000000000000000 ) ) ;
#5317=ADVANCED_FACE ( 'NONE', ( #6483 ), #7832, .T. ) ;
#5321=CARTESIAN_POINT ( 'NONE',  ( 3.200012235603504143E-34, -50.00000000000008527, 130.0000000000000000 ) ) ;
#5332=VERTEX_POINT ( 'NONE', #3750 ) ;
#5333=CARTESIAN_POINT ( 'NONE',  ( -28.24999999999997513, 3.989921841591238568E-15, -6.938893903907228378E-15 ) ) ;
#5337=DIRECTION ( 'NONE',  ( 6.400024471206997542E-36, -1.000000000000000000, 0.000000000000000000 ) ) ;
#5339=CIRCLE ( 'NONE', #2271, 40.00000000000007816 ) ;
#5359=EDGE_CURVE ( 'NONE', #5332, #2816, #4521, .T. ) ;
#5380=EDGE_CURVE ( 'NONE', #7854, #4358, #7166, .T. ) ;
#5386=CIRCLE ( 'NONE', #1199, 4.250000000000010658 ) ;
#5420=AXIS2_PLACEMENT_3D ( 'NONE', #7518, #2241, #1542 ) ;
#5422=ORIENTED_EDGE ( 'NONE', *, *, #8604, .F. ) ;
#5441=CARTESIAN_POINT ( 'NONE',  ( 0.000000000000000000, 0.000000000000000000, 18.00000000000000355 ) ) ;
#5455=CARTESIAN_POINT ( 'NONE',  ( 6.123233995736776340E-15, 50.00000000000008527, 130.0000000000000000 ) ) ;
#5468=ORIENTED_EDGE ( 'NONE', *, *, #2831, .F. ) ;
#5471=VERTEX_POINT ( 'NONE', #6437 ) ;
#5474=DIRECTION ( 'NONE',  ( 0.7071067811865456854, 8.659560562354910671E-17, -0.7071067811865493491 ) ) ;
#5486=CARTESIAN_POINT ( 'NONE',  ( -28.24999999999996447, 3.989921841591239357E-15, 18.00000000000000355 ) ) ;
#5487=VECTOR ( 'NONE', #7411, 1000.000000000000000 ) ;
#5499=CARTESIAN_POINT ( 'NONE',  ( -1.954730054507676012E-32, 40.00000000000000711, 3.039269428540889921E-16 ) ) ;
#5506=SHAPE_REPRESENTATION ( 'Servo motor', ( #7563 ), #6881 ) ;
#5508=( NAMED_UNIT ( * ) SI_UNIT ( $, .STERADIAN. ) SOLID_ANGLE_UNIT ( ) );
#5525=CARTESIAN_POINT ( 'NONE',  ( 5.510910596163089556E-15, -40.00000000000000711, -3.039269428540889921E-16 ) ) ;
#5538=FACE_OUTER_BOUND ( 'NONE', #7016, .T. ) ;
#5539=ORIENTED_EDGE ( 'NONE', *, *, #3193, .F. ) ;
#5541=PLANE ( 'NONE',  #3241 ) ;
#5543=CYLINDRICAL_SURFACE ( 'NONE', #812, 4.250000000000003553 ) ;
#5544=ORIENTED_EDGE ( 'NONE', *, *, #2789, .F. ) ;
#5546=VECTOR ( 'NONE', #352, 1000.000000000000000 ) ;
#5565=CARTESIAN_POINT ( 'NONE',  ( 4.250000000000008882, 32.50000000000005684, 18.00000000000000355 ) ) ;
#5587=DIRECTION ( 'NONE',  ( 3.851859888774471706E-33, 1.232595164407830946E-32, 1.000000000000000000 ) ) ;
#5618=( NAMED_UNIT ( * ) PLANE_ANGLE_UNIT ( ) SI_UNIT ( $, .RADIAN. ) );
#5633=CARTESIAN_POINT ( 'NONE',  ( 32.49999999999997158, 1.387778780781445676E-14, 18.00000000000000355 ) ) ;
#5634=ORIENTED_EDGE ( 'NONE', *, *, #245, .F. ) ;
#5661=APPLICATION_CONTEXT ( 'automotive_design' ) ;
#5663=CARTESIAN_POINT ( 'NONE',  ( -15.00000000000000000, -1.111739529205948433E-31, 6.018531076210101093E-32 ) ) ;
#5670=CARTESIAN_POINT ( 'NONE',  ( 0.000000000000000000, -1.040834085586084257E-14, -120.0000000000000000 ) ) ;
#5672=DIRECTION ( 'NONE',  ( -3.851859888774471706E-33, -1.232595164407830946E-32, -1.000000000000000000 ) ) ;
#5674=ADVANCED_FACE ( 'NONE', ( #1905 ), #6657, .T. ) ;
#5688=DIRECTION ( 'NONE',  ( -3.851859888774471706E-33, -1.232595164407830946E-32, -1.000000000000000000 ) ) ;
#5690=AXIS2_PLACEMENT_3D ( 'NONE', #1403, #4139, #7456 ) ;
#5692=DIRECTION ( 'NONE',  ( -3.851859888774471706E-33, 7.598173571352223877E-18, -1.000000000000000000 ) ) ;
#5693=AXIS2_PLACEMENT_3D ( 'NONE', #4562, #3955, #5975 ) ;
#5695=CARTESIAN_POINT ( 'NONE',  ( 0.000000000000000000, -3.469446951953614189E-15, 128.9999999999999432 ) ) ;
#5721=FACE_OUTER_BOUND ( 'NONE', #6959, .T. ) ;
#5724=CYLINDRICAL_SURFACE ( 'NONE', #7285, 4.250000000000014211 ) ;
#5728=ADVANCED_FACE ( 'NONE', ( #3495 ), #3315, .T. ) ;
#5730=MANIFOLD_SOLID_BREP ( 'Chamfer2', #4874 ) ;
#5754=ORIENTED_EDGE ( 'NONE', *, *, #6591, .T. ) ;
#5757=DIRECTION ( 'NONE',  ( 2.728201748236233471E-33, -0.7071067811865491270, 0.7071067811865459074 ) ) ;
#5761=AXIS2_PLACEMENT_3D ( 'NONE', #6355, #8220, #7482 ) ;
#5773=DIRECTION ( 'NONE',  ( 3.851859888774471706E-33, -7.598173571352216173E-18, 1.000000000000000000 ) ) ;
#5778=AXIS2_PLACEMENT_3D ( 'NONE', #6852, #7502, #2057 ) ;
#5780=CONICAL_SURFACE ( 'NONE', #1707, 38.74999999999999289, 0.7853981633974447263 ) ;
#5792=CARTESIAN_POINT ( 'NONE',  ( 0.000000000000000000, 0.000000000000000000, -10.00000000000006395 ) ) ;
#5799=CARTESIAN_POINT ( 'NONE',  ( 6.123233995736764507E-15, 49.99999999999999289, -109.9999999999999574 ) ) ;
#5803=DIRECTION ( 'NONE',  ( -1.000000000000000000, 0.000000000000000000, 0.000000000000000000 ) ) ;
#5811=VERTEX_POINT ( 'NONE', #2085 ) ;
#5823=CARTESIAN_POINT ( 'NONE',  ( 0.000000000000000000, -3.469446951953614189E-15, 130.0000000000000000 ) ) ;
#5825=VERTEX_POINT ( 'NONE', #1907 ) ;
#5833=LINE ( 'NONE', #667, #425 ) ;
#5846=PLANE ( 'NONE',  #3102 ) ;
#5861=CIRCLE ( 'NONE', #3325, 4.250000000000006217 ) ;
#5871=CIRCLE ( 'NONE', #2100, 4.250000000000007105 ) ;
#5878=ORIENTED_EDGE ( 'NONE', *, *, #3401, .F. ) ;
#5883=ORIENTED_EDGE ( 'NONE', *, *, #7319, .F. ) ;
#5891=DIRECTION ( 'NONE',  ( 6.400024471206996205E-36, -1.000000000000000000, -7.598173571352216173E-18 ) ) ;
#5900=EDGE_LOOP ( 'NONE', ( #906, #4736 ) ) ;
#5918=AXIS2_PLACEMENT_3D ( 'NONE', #8512, #2514, #3740 ) ;
#5924=DIRECTION ( 'NONE',  ( -3.851859888774471706E-33, -1.232595164407830946E-32, -1.000000000000000000 ) ) ;
#5928=EDGE_CURVE ( 'NONE', #7472, #7867, #5250, .T. ) ;
#5940=DIRECTION ( 'NONE',  ( 3.851859888774471706E-33, -7.598173571352220795E-18, 1.000000000000000000 ) ) ;
#5944=EDGE_LOOP ( 'NONE', ( #1500, #68, #946, #4514 ) ) ;
#5946=DIRECTION ( 'NONE',  ( 6.400024471206993532E-36, -1.000000000000000000, -7.598173571352213092E-18 ) ) ;
#5949=ADVANCED_BREP_SHAPE_REPRESENTATION ( '', ( #5730, #7563 ), #6881 ) ;
#5954=CARTESIAN_POINT ( 'NONE',  ( 32.49999999999997158, 1.387778780781445676E-14, 18.00000000000000355 ) ) ;
#5960=EDGE_CURVE ( 'NONE', #3289, #5332, #4029, .T. ) ;
#5965=CARTESIAN_POINT ( 'NONE',  ( 0.000000000000000000, -3.469446951953614189E-15, 130.0000000000000000 ) ) ;
#5968=ORIENTED_EDGE ( 'NONE', *, *, #4528, .F. ) ;
#5969=EDGE_CURVE ( 'NONE', #2630, #7000, #1798, .T. ) ;
#5975=DIRECTION ( 'NONE',  ( -1.000000000000000000, 1.284024588418159817E-35, 0.000000000000000000 ) ) ;
#6005=EDGE_CURVE ( 'NONE', #6260, #7754, #4649, .T. ) ;
#6017=DIRECTION ( 'NONE',  ( -3.851859888774471706E-33, -1.232595164407830946E-32, -1.000000000000000000 ) ) ;
#6026=ORIENTED_EDGE ( 'NONE', *, *, #5180, .T. ) ;
#6028=VERTEX_POINT ( 'NONE', #6059 ) ;
#6033=ADVANCED_FACE ( 'NONE', ( #4602 ), #8041, .T. ) ;
#6047=VECTOR ( 'NONE', #8137, 1000.000000000000000 ) ;
#6050=VECTOR ( 'NONE', #6713, 1000.000000000000000 ) ;
#6059=CARTESIAN_POINT ( 'NONE',  ( 1.224646799147351679E-15, -9.499999999999984013, 130.0000000000000000 ) ) ;
#6089=CARTESIAN_POINT ( 'NONE',  ( 36.74999999999998579, 1.439826269745208429E-14, 18.00000000000000355 ) ) ;
#6111=ORIENTED_EDGE ( 'NONE', *, *, #1704, .T. ) ;
#6112=DIRECTION ( 'NONE',  ( 3.851859888774471706E-33, 1.232595164407830946E-32, 1.000000000000000000 ) ) ;
#6121=ORIENTED_EDGE ( 'NONE', *, *, #7719, .T. ) ;
#6125=AXIS2_PLACEMENT_3D ( 'NONE', #5035, #8471, #545 ) ;
#6134=AXIS2_PLACEMENT_3D ( 'NONE', #6225, #2894, #283 ) ;
#6164=CARTESIAN_POINT ( 'NONE',  ( -36.74999999999997868, 3.469446951953614189E-15, 18.00000000000000355 ) ) ;
#6177=AXIS2_PLACEMENT_3D ( 'NONE', #6597, #8080, #7379 ) ;
#6178=ORIENTED_EDGE ( 'NONE', *, *, #4473, .T. ) ;
#6187=ORIENTED_EDGE ( 'NONE', *, *, #7344, .T. ) ;
#6188=CIRCLE ( 'NONE', #5778, 4.250000000000008882 ) ;
#6199=CARTESIAN_POINT ( 'NONE',  ( -32.49999999999997158, 3.469446951953614189E-15, 18.00000000000000355 ) ) ;
#6209=ORIENTED_EDGE ( 'NONE', *, *, #875, .T. ) ;
#6219=EDGE_LOOP ( 'NONE', ( #1123, #5292, #6121, #1367 ) ) ;
#6225=CARTESIAN_POINT ( 'NONE',  ( 0.000000000000000000, 32.50000000000005684, 18.00000000000000355 ) ) ;
#6242=FACE_OUTER_BOUND ( 'NONE', #4547, .T. ) ;
#6247=ORIENTED_EDGE ( 'NONE', *, *, #7924, .F. ) ;
#6254=ADVANCED_FACE ( 'NONE', ( #6453 ), #12, .T. ) ;
#6256=CYLINDRICAL_SURFACE ( 'NONE', #4164, 4.250000000000008882 ) ;
#6260=VERTEX_POINT ( 'NONE', #7063 ) ;
#6275=VECTOR ( 'NONE', #8259, 1000.000000000000227 ) ;
#6298=DIRECTION ( 'NONE',  ( 6.400024471206996205E-36, -1.000000000000000000, -7.598173571352216173E-18 ) ) ;
#6324=CARTESIAN_POINT ( 'NONE',  ( -39.75000000000007105, 5.103997738962193686E-34, 18.00000000000000355 ) ) ;
#6332=CARTESIAN_POINT ( 'NONE',  ( 0.000000000000000000, -32.50000000000004974, 18.00000000000000355 ) ) ;
#6335=DIRECTION ( 'NONE',  ( -3.851859888774471706E-33, -1.232595164407830946E-32, -1.000000000000000000 ) ) ;
#6340=CARTESIAN_POINT ( 'NONE',  ( 0.000000000000000000, 0.000000000000000000, 0.000000000000000000 ) ) ;
#6355=CARTESIAN_POINT ( 'NONE',  ( 0.000000000000000000, 0.000000000000000000, 18.00000000000000355 ) ) ;
#6357=VERTEX_POINT ( 'NONE', #2576 ) ;
#6368=CARTESIAN_POINT ( 'NONE',  ( 0.000000000000000000, 0.000000000000000000, 18.00000000000000355 ) ) ;
#6397=DIRECTION ( 'NONE',  ( 3.851859888774471706E-33, 1.232595164407830946E-32, 1.000000000000000000 ) ) ;
#6412=AXIS2_PLACEMENT_3D ( 'NONE', #1945, #595, #3743 ) ;
#6415=EDGE_CURVE ( 'NONE', #4181, #7660, #3451, .T. ) ;
#6437=CARTESIAN_POINT ( 'NONE',  ( -4.250000000000000888, -32.50000000000004974, 18.00000000000000355 ) ) ;
#6446=ORIENTED_EDGE ( 'NONE', *, *, #2756, .F. ) ;
#6447=EDGE_LOOP ( 'NONE', ( #5468, #3166 ) ) ;
#6453=FACE_OUTER_BOUND ( 'NONE', #6811, .T. ) ;
#6457=DIRECTION ( 'NONE',  ( 1.000000000000000000, 0.000000000000000000, 0.000000000000000000 ) ) ;
#6463=CARTESIAN_POINT ( 'NONE',  ( 3.200012235603505854E-34, -50.00000000000008527, -10.00000000000006395 ) ) ;
#6483=FACE_OUTER_BOUND ( 'NONE', #2456, .T. ) ;
#6490=ORIENTED_EDGE ( 'NONE', *, *, #1794, .T. ) ;
#6496=DIRECTION ( 'NONE',  ( -3.851859888774471706E-33, 7.598173571352185358E-18, -1.000000000000000000 ) ) ;
#6512=FACE_OUTER_BOUND ( 'NONE', #311, .T. ) ;
#6525=DIRECTION ( 'NONE',  ( 3.851859888774471706E-33, -7.598173571352223877E-18, 1.000000000000000000 ) ) ;
#6527=CIRCLE ( 'NONE', #6134, 4.250000000000008882 ) ;
#6530=ORIENTED_EDGE ( 'NONE', *, *, #2143, .T. ) ;
#6591=EDGE_CURVE ( 'NONE', #5825, #2630, #4962, .T. ) ;
#6597=CARTESIAN_POINT ( 'NONE',  ( 0.000000000000000000, 0.000000000000000000, 18.00000000000000355 ) ) ;
#6602=ADVANCED_FACE ( 'NONE', ( #1565 ), #5543, .F. ) ;
#6607=ORIENTED_EDGE ( 'NONE', *, *, #3879, .T. ) ;
#6647=CARTESIAN_POINT ( 'NONE',  ( 0.000000000000000000, 0.000000000000000000, 16.99999999999991829 ) ) ;
#6656=ADVANCED_FACE ( 'NONE', ( #3710 ), #6934, .F. ) ;
#6657=PLANE ( 'NONE',  #2740 ) ;
#6681=DIRECTION ( 'NONE',  ( 6.400024471207029615E-36, -1.000000000000000000, 0.000000000000000000 ) ) ;
#6688=ORIENTED_EDGE ( 'NONE', *, *, #8604, .T. ) ;
#6692=CARTESIAN_POINT ( 'NONE',  ( 15.00000000000002487, 1.836970198721033139E-15, 18.00000000000000355 ) ) ;
#6713=DIRECTION ( 'NONE',  ( 3.851859888774471706E-33, -7.598173571352223877E-18, 1.000000000000000000 ) ) ;
#6721=AXIS2_PLACEMENT_3D ( 'NONE', #2320, #4333, #1028 ) ;
#6738=VECTOR ( 'NONE', #4556, 1000.000000000000000 ) ;
#6759=ORIENTED_EDGE ( 'NONE', *, *, #7319, .T. ) ;
#6760=CARTESIAN_POINT ( 'NONE',  ( 0.000000000000000000, -32.50000000000004974, 18.00000000000000355 ) ) ;
#6767=CARTESIAN_POINT ( 'NONE',  ( -4.250000000000000888, 32.50000000000005684, 18.00000000000000355 ) ) ;
#6783=ORIENTED_EDGE ( 'NONE', *, *, #3725, .F. ) ;
#6785=ADVANCED_FACE ( 'NONE', ( #1207 ), #518, .T. ) ;
#6797=DIRECTION ( 'NONE',  ( 6.400024471206996205E-36, -1.000000000000000000, -7.598173571352216173E-18 ) ) ;
#6802=ADVANCED_FACE ( 'NONE', ( #7876 ), #3084, .T. ) ;
#6805=CARTESIAN_POINT ( 'NONE',  ( 4.250000000000000888, -32.50000000000004974, 18.00000000000000355 ) ) ;
#6809=ORIENTED_EDGE ( 'NONE', *, *, #7924, .T. ) ;
#6811=EDGE_LOOP ( 'NONE', ( #8186, #6446, #2712, #7014 ) ) ;
#6831=VECTOR ( 'NONE', #1575, 1000.000000000000000 ) ;
#6841=ORIENTED_EDGE ( 'NONE', *, *, #6591, .F. ) ;
#6852=CARTESIAN_POINT ( 'NONE',  ( 0.000000000000000000, -32.50000000000004974, 18.00000000000000355 ) ) ;
#6866=CIRCLE ( 'NONE', #4633, 50.00000000000008527 ) ;
#6881=( GEOMETRIC_REPRESENTATION_CONTEXT ( 3 ) GLOBAL_UNCERTAINTY_ASSIGNED_CONTEXT ( ( #3051 ) ) GLOBAL_UNIT_ASSIGNED_CONTEXT ( ( #945, #5618, #4291 ) ) REPRESENTATION_CONTEXT ( 'NONE', 'WORKASPACE' ) );
#6891=CARTESIAN_POINT ( 'NONE',  ( 0.000000000000000000, 0.000000000000000000, 0.000000000000000000 ) ) ;
#6901=DIRECTION ( 'NONE',  ( -3.851859888774471706E-33, -1.232595164407830946E-32, -1.000000000000000000 ) ) ;
#6903=EDGE_LOOP ( 'NONE', ( #3252, #42, #6530, #8373 ) ) ;
#6913=CIRCLE ( 'NONE', #505, 39.75000000000007105 ) ;
#6934=CYLINDRICAL_SURFACE ( 'NONE', #4567, 4.250000000000008882 ) ;
#6953=LINE ( 'NONE', #8085, #226 ) ;
#6959=EDGE_LOOP ( 'NONE', ( #8555, #6809, #4075, #5539 ) ) ;
#6990=DIRECTION ( 'NONE',  ( 3.851859888774471706E-33, 1.232595164407830946E-32, 1.000000000000000000 ) ) ;
#6991=CARTESIAN_POINT ( 'NONE',  ( -39.75000000000000000, -1.165861408448480429E-31, 1.925929944387232350E-31 ) ) ;
#6999=DIRECTION ( 'NONE',  ( 3.851859888774471706E-33, -7.598173571352223877E-18, 1.000000000000000000 ) ) ;
#7000=VERTEX_POINT ( 'NONE', #4303 ) ;
#7004=ORIENTED_EDGE ( 'NONE', *, *, #7171, .T. ) ;
#7005=CARTESIAN_POINT ( 'NONE',  ( 6.720025694767360582E-35, -10.50000000000002132, -7.978082249919844238E-17 ) ) ;
#7006=PRODUCT_DEFINITION_CONTEXT ( 'detailed design', #7856, 'design' ) ;
#7014=ORIENTED_EDGE ( 'NONE', *, *, #4710, .F. ) ;
#7015=CARTESIAN_POINT ( 'NONE',  ( -4.250000000000000888, -32.50000000000004974, 1.504632769052525000E-32 ) ) ;
#7016=EDGE_LOOP ( 'NONE', ( #4356, #2893 ) ) ;
#7026=CARTESIAN_POINT ( 'NONE',  ( 0.000000000000000000, -1.387778780781445676E-14, -120.0000000000000000 ) ) ;
#7030=AXIS2_PLACEMENT_3D ( 'NONE', #1733, #5692, #3134 ) ;
#7039=ORIENTED_EDGE ( 'NONE', *, *, #5380, .T. ) ;
#7051=ORIENTED_EDGE ( 'NONE', *, *, #2072, .F. ) ;
#7052=CIRCLE ( 'NONE', #1488, 38.74999999999999289 ) ;
#7053=DIRECTION ( 'NONE',  ( 1.000000000000000000, -1.284024588418159550E-35, 0.000000000000000000 ) ) ;
#7056=DIRECTION ( 'NONE',  ( -3.851859888774471706E-33, 7.598173571352223877E-18, -1.000000000000000000 ) ) ;
#7063=CARTESIAN_POINT ( 'NONE',  ( 15.00000000000000000, 1.836970198721029589E-15, 18.00000000000000355 ) ) ;
#7067=AXIS2_PLACEMENT_3D ( 'NONE', #939, #4286, #8212 ) ;
#7080=CARTESIAN_POINT ( 'NONE',  ( 3.200012235603505426E-34, -50.00000000000008527, -109.9999999999999574 ) ) ;
#7099=DIRECTION ( 'NONE',  ( 6.400024471206996205E-36, -1.000000000000000000, -7.598173571352216173E-18 ) ) ;
#7100=( GEOMETRIC_REPRESENTATION_CONTEXT ( 3 ) GLOBAL_UNCERTAINTY_ASSIGNED_CONTEXT ( ( #7670 ) ) GLOBAL_UNIT_ASSIGNED_CONTEXT ( ( #1319, #2056, #5508 ) ) REPRESENTATION_CONTEXT ( 'NONE', 'WORKASPACE' ) );
#7105=VECTOR ( 'NONE', #6017, 1000.000000000000000 ) ;
#7161=ORIENTED_EDGE ( 'NONE', *, *, #7171, .F. ) ;
#7166=CIRCLE ( 'NONE', #7030, 4.250000000000006217 ) ;
#7171=EDGE_CURVE ( 'NONE', #5811, #3646, #115, .T. ) ;
#7241=CARTESIAN_POINT ( 'NONE',  ( 0.000000000000000000, -3.469446951953614189E-15, 128.9999999999999432 ) ) ;
#7252=DIRECTION ( 'NONE',  ( 0.000000000000000000, -1.000000000000000000, -7.598173571352217714E-18 ) ) ;
#7266=VECTOR ( 'NONE', #7772, 1000.000000000000227 ) ;
#7277=VECTOR ( 'NONE', #8111, 1000.000000000000000 ) ;
#7282=LINE ( 'NONE', #6164, #5487 ) ;
#7285=AXIS2_PLACEMENT_3D ( 'NONE', #5633, #4872, #2180 ) ;
#7293=CYLINDRICAL_SURFACE ( 'NONE', #6177, 15.00000000000002487 ) ;
#7312=DIRECTION ( 'NONE',  ( 3.851859888774471706E-33, -7.598173571352223877E-18, 1.000000000000000000 ) ) ;
#7315=ORIENTED_EDGE ( 'NONE', *, *, #8404, .F. ) ;
#7319=EDGE_CURVE ( 'NONE', #6028, #7472, #3628, .T. ) ;
#7325=ORIENTED_EDGE ( 'NONE', *, *, #3031, .F. ) ;
#7340=DIRECTION ( 'NONE',  ( -3.851859888774471706E-33, -1.232595164407830946E-32, -1.000000000000000000 ) ) ;
#7344=EDGE_CURVE ( 'NONE', #1987, #7754, #7364, .T. ) ;
#7358=AXIS2_PLACEMENT_3D ( 'NONE', #7720, #3064, #3803 ) ;
#7361=AXIS2_PLACEMENT_3D ( 'NONE', #2243, #1501, #4899 ) ;
#7364=CIRCLE ( 'NONE', #2088, 15.00000000000002487 ) ;
#7370=CIRCLE ( 'NONE', #3627, 4.250000000000008882 ) ;
#7376=EDGE_CURVE ( 'NONE', #3646, #5811, #4310, .T. ) ;
#7379=DIRECTION ( 'NONE',  ( -1.000000000000000000, 1.284024588418159817E-35, 0.000000000000000000 ) ) ;
#7411=DIRECTION ( 'NONE',  ( -3.851859888774471706E-33, -1.232595164407830946E-32, -1.000000000000000000 ) ) ;
#7414=EDGE_CURVE ( 'NONE', #3572, #7660, #2491, .T. ) ;
#7422=CARTESIAN_POINT ( 'NONE',  ( 0.000000000000000000, 32.50000000000005684, 18.00000000000000355 ) ) ;
#7430=CARTESIAN_POINT ( 'NONE',  ( -4.250000000000008882, 32.50000000000005684, 18.00000000000000355 ) ) ;
#7456=DIRECTION ( 'NONE',  ( 6.400024471207000214E-36, -1.000000000000000000, 0.000000000000000000 ) ) ;
#7457=EDGE_CURVE ( 'NONE', #922, #4232, #6527, .T. ) ;
#7471=VERTEX_POINT ( 'NONE', #5525 ) ;
#7472=VERTEX_POINT ( 'NONE', #8171 ) ;
#7478=DIRECTION ( 'NONE',  ( 0.000000000000000000, 0.000000000000000000, 1.000000000000000000 ) ) ;
#7482=DIRECTION ( 'NONE',  ( -1.000000000000000000, 1.284024588418159550E-35, 0.000000000000000000 ) ) ;
#7492=EDGE_CURVE ( 'NONE', #4232, #4496, #2204, .T. ) ;
#7494=DIRECTION ( 'NONE',  ( -1.000000000000000000, 1.284024588418159550E-35, 0.000000000000000000 ) ) ;
#7502=DIRECTION ( 'NONE',  ( 3.851859888774471706E-33, 1.232595164407830946E-32, 1.000000000000000000 ) ) ;
#7509=ORIENTED_EDGE ( 'NONE', *, *, #6005, .F. ) ;
#7512=CIRCLE ( 'NONE', #979, 4.250000000000008882 ) ;
#7514=CARTESIAN_POINT ( 'NONE',  ( 3.200012235603505426E-34, -50.00000000000008527, -109.9999999999999574 ) ) ;
#7518=CARTESIAN_POINT ( 'NONE',  ( -32.49999999999997158, 3.469446951953614189E-15, 18.00000000000000355 ) ) ;
#7521=EDGE_CURVE ( 'NONE', #7819, #3380, #4819, .T. ) ;
#7529=DIRECTION ( 'NONE',  ( 3.851859888774471706E-33, -7.598173571352220795E-18, 1.000000000000000000 ) ) ;
#7537=CARTESIAN_POINT ( 'NONE',  ( 0.000000000000000000, 0.000000000000000000, 18.00000000000000355 ) ) ;
#7563=AXIS2_PLACEMENT_3D ( 'NONE', #4203, #7478, #3512 ) ;
#7567=AXIS2_PLACEMENT_3D ( 'NONE', #4879, #169, #3665 ) ;
#7589=LINE ( 'NONE', #6089, #4034 ) ;
#7607=DIRECTION ( 'NONE',  ( 6.400024471206997542E-36, -1.000000000000000000, 0.000000000000000000 ) ) ;
#7641=ORIENTED_EDGE ( 'NONE', *, *, #4946, .F. ) ;
#7652=DIRECTION ( 'NONE',  ( 1.000000000000000000, -1.284024588418159550E-35, 3.851859888774464864E-33 ) ) ;
#7660=VERTEX_POINT ( 'NONE', #6463 ) ;
#7663=ORIENTED_EDGE ( 'NONE', *, *, #394, .T. ) ;
#7670=UNCERTAINTY_MEASURE_WITH_UNIT (LENGTH_MEASURE( 1.000000000000000082E-05 ), #1319, 'distance_accuracy_value', 'NONE');
#7676=CARTESIAN_POINT ( 'NONE',  ( 32.49999999999997158, 1.387778780781445676E-14, 18.00000000000000355 ) ) ;
#7684=VERTEX_POINT ( 'NONE', #1664 ) ;
#7690=FACE_OUTER_BOUND ( 'NONE', #1226, .T. ) ;
#7701=AXIS2_PLACEMENT_3D ( 'NONE', #3564, #241, #775 ) ;
#7703=CIRCLE ( 'NONE', #8263, 39.75000000000007105 ) ;
#7706=ORIENTED_EDGE ( 'NONE', *, *, #6415, .T. ) ;
#7719=EDGE_CURVE ( 'NONE', #5471, #2816, #5833, .T. ) ;
#7720=CARTESIAN_POINT ( 'NONE',  ( 0.000000000000000000, 0.000000000000000000, 18.00000000000000355 ) ) ;
#7721=EDGE_LOOP ( 'NONE', ( #7161, #295 ) ) ;
#7746=ORIENTED_EDGE ( 'NONE', *, *, #4375, .T. ) ;
#7754=VERTEX_POINT ( 'NONE', #43 ) ;
#7771=CONICAL_SURFACE ( 'NONE', #981, 40.00000000000007816, 0.7853981633974445042 ) ;
#7772=DIRECTION ( 'NONE',  ( 8.659560562354906974E-17, -0.7071067811865454633, -0.7071067811865495711 ) ) ;
#7814=VECTOR ( 'NONE', #8017, 1000.000000000000000 ) ;
#7818=DIRECTION ( 'NONE',  ( 3.851859888774471706E-33, -7.598173571352216173E-18, 1.000000000000000000 ) ) ;
#7819=VERTEX_POINT ( 'NONE', #4637 ) ;
#7832=CYLINDRICAL_SURFACE ( 'NONE', #1052, 10.50000000000001066 ) ;
#7849=ORIENTED_EDGE ( 'NONE', *, *, #2951, .F. ) ;
#7854=VERTEX_POINT ( 'NONE', #5333 ) ;
#7856=APPLICATION_CONTEXT ( 'automotive_design' ) ;
#7863=FACE_OUTER_BOUND ( 'NONE', #8180, .T. ) ;
#7867=VERTEX_POINT ( 'NONE', #1492 ) ;
#7871=FACE_OUTER_BOUND ( 'NONE', #1667, .T. ) ;
#7876=FACE_OUTER_BOUND ( 'NONE', #3560, .T. ) ;
#7880=ORIENTED_EDGE ( 'NONE', *, *, #1222, .T. ) ;
#7894=CARTESIAN_POINT ( 'NONE',  ( 4.250000000000000888, 32.50000000000005684, -6.938893903907228378E-15 ) ) ;
#7900=EDGE_LOOP ( 'NONE', ( #1625, #8515, #422, #2109 ) ) ;
#7922=DIRECTION ( 'NONE',  ( 1.000000000000000000, -1.284024588418159550E-35, 3.851859888774464864E-33 ) ) ;
#7924=EDGE_CURVE ( 'NONE', #2093, #3646, #7589, .T. ) ;
#7942=ORIENTED_EDGE ( 'NONE', *, *, #4325, .T. ) ;
#7971=EDGE_LOOP ( 'NONE', ( #3804, #3082, #2586, #3523 ) ) ;
#7984=DIRECTION ( 'NONE',  ( 3.851859888774471706E-33, -7.598173571352223877E-18, 1.000000000000000000 ) ) ;
#8007=DIRECTION ( 'NONE',  ( 6.400024471207000214E-36, -1.000000000000000000, 0.000000000000000000 ) ) ;
#8017=DIRECTION ( 'NONE',  ( -3.851859888774471706E-33, -1.232595164407830946E-32, -1.000000000000000000 ) ) ;
#8022=EDGE_CURVE ( 'NONE', #3886, #749, #8201, .T. ) ;
#8036=CARTESIAN_POINT ( 'NONE',  ( 6.123233995736764507E-15, 49.99999999999999289, -10.00000000000006395 ) ) ;
#8038=CARTESIAN_POINT ( 'NONE',  ( 28.24999999999996803, 1.387778780781445676E-14, 18.00000000000000355 ) ) ;
#8041=CYLINDRICAL_SURFACE ( 'NONE', #2383, 50.00000000000008527 ) ;
#8042=DIRECTION ( 'NONE',  ( 3.851859888774471706E-33, -7.598173571352223877E-18, 1.000000000000000000 ) ) ;
#8048=EDGE_CURVE ( 'NONE', #2093, #4094, #431, .T. ) ;
#8052=CIRCLE ( 'NONE', #279, 10.50000000000001066 ) ;
#8080=DIRECTION ( 'NONE',  ( -3.851859888774471706E-33, -1.232595164407830946E-32, -1.000000000000000000 ) ) ;
#8084=ADVANCED_FACE ( 'NONE', ( #8374 ), #7771, .T. ) ;
#8085=CARTESIAN_POINT ( 'NONE',  ( 38.74999999999999289, 4.745506346695993302E-15, 18.00000000000000355 ) ) ;
#8088=CARTESIAN_POINT ( 'NONE',  ( 6.123233995736776340E-15, 50.00000000000008527, -109.9999999999999574 ) ) ;
#8109=DIRECTION ( 'NONE',  ( -2.728201748236247839E-33, 0.7071067811865454633, -0.7071067811865495711 ) ) ;
#8111=DIRECTION ( 'NONE',  ( 3.851859888774471706E-33, -7.598173571352223877E-18, 1.000000000000000000 ) ) ;
#8124=ORIENTED_EDGE ( 'NONE', *, *, #3401, .T. ) ;
#8137=DIRECTION ( 'NONE',  ( -3.851859888774471706E-33, -1.232595164407830946E-32, -1.000000000000000000 ) ) ;
#8149=DIRECTION ( 'NONE',  ( -3.851859888774471706E-33, -1.232595164407830946E-32, -1.000000000000000000 ) ) ;
#8171=CARTESIAN_POINT ( 'NONE',  ( -1.989930189099410700E-33, 9.499999999999976907, 130.0000000000000000 ) ) ;
#8177=DIRECTION ( 'NONE',  ( 6.400024471207000214E-36, -1.000000000000000000, 0.000000000000000000 ) ) ;
#8180=EDGE_LOOP ( 'NONE', ( #3536, #6688, #1349, #1248 ) ) ;
#8182=ORIENTED_EDGE ( 'NONE', *, *, #7414, .T. ) ;
#8186=ORIENTED_EDGE ( 'NONE', *, *, #710, .F. ) ;
#8201=LINE ( 'NONE', #4887, #6831 ) ;
#8205=DIRECTION ( 'NONE',  ( 3.851859888774471706E-33, 1.232595164407830946E-32, 1.000000000000000000 ) ) ;
#8210=CARTESIAN_POINT ( 'NONE',  ( 6.720025694767387310E-35, -10.50000000000001421, 128.9999999999999432 ) ) ;
#8212=DIRECTION ( 'NONE',  ( -6.400024471207028278E-36, 1.000000000000000000, 0.000000000000000000 ) ) ;
#8217=ORIENTED_EDGE ( 'NONE', *, *, #2537, .T. ) ;
#8220=DIRECTION ( 'NONE',  ( -3.851859888774471706E-33, -1.232595164407830946E-32, -1.000000000000000000 ) ) ;
#8232=DIRECTION ( 'NONE',  ( 3.851859888774471706E-33, 1.232595164407830946E-32, 1.000000000000000000 ) ) ;
#8233=ORIENTED_EDGE ( 'NONE', *, *, #3929, .F. ) ;
#8257=ORIENTED_EDGE ( 'NONE', *, *, #1592, .F. ) ;
#8259=DIRECTION ( 'NONE',  ( 8.659560562354952580E-17, 0.7071067811865491270, 0.7071067811865459074 ) ) ;
#8263=AXIS2_PLACEMENT_3D ( 'NONE', #1334, #7340, #3988 ) ;
#8275=CARTESIAN_POINT ( 'NONE',  ( 0.000000000000000000, 0.000000000000000000, 0.000000000000000000 ) ) ;
#8280=FACE_BOUND ( 'NONE', #3444, .T. ) ;
#8295=FACE_OUTER_BOUND ( 'NONE', #3674, .T. ) ;
#8318=DIRECTION ( 'NONE',  ( 3.851859888774471706E-33, -7.598173571352216173E-18, 1.000000000000000000 ) ) ;
#8340=VERTEX_POINT ( 'NONE', #4261 ) ;
#8346=AXIS2_PLACEMENT_3D ( 'NONE', #2770, #8042, #1374 ) ;
#8370=EDGE_CURVE ( 'NONE', #4915, #7471, #2410, .T. ) ;
#8373=ORIENTED_EDGE ( 'NONE', *, *, #8022, .F. ) ;
#8374=FACE_OUTER_BOUND ( 'NONE', #7971, .T. ) ;
#8378=ADVANCED_FACE ( 'NONE', ( #2335 ), #5724, .F. ) ;
#8382=CIRCLE ( 'NONE', #4631, 4.250000000000010658 ) ;
#8404=EDGE_CURVE ( 'NONE', #2630, #2559, #1003, .T. ) ;
#8409=DIRECTION ( 'NONE',  ( -3.851859888774471706E-33, 7.598173571352223877E-18, -1.000000000000000000 ) ) ;
#8421=AXIS2_PLACEMENT_3D ( 'NONE', #4527, #8409, #2436 ) ;
#8424=ADVANCED_FACE ( 'NONE', ( #7863 ), #1768, .T. ) ;
#8471=DIRECTION ( 'NONE',  ( -3.851859888774471706E-33, 7.598173571352223877E-18, -1.000000000000000000 ) ) ;
#8490=ORIENTED_EDGE ( 'NONE', *, *, #5969, .F. ) ;
#8503=VECTOR ( 'NONE', #721, 1000.000000000000000 ) ;
#8512=CARTESIAN_POINT ( 'NONE',  ( 0.000000000000000000, 0.000000000000000000, 18.00000000000000355 ) ) ;
#8515=ORIENTED_EDGE ( 'NONE', *, *, #7492, .T. ) ;
#8519=ADVANCED_FACE ( 'NONE', ( #6512, #511 ), #5846, .T. ) ;
#8536=EDGE_LOOP ( 'NONE', ( #790, #2886 ) ) ;
#8544=PRODUCT_DEFINITION_SHAPE ( 'NONE', 'NONE',  #297 ) ;
#8555=ORIENTED_EDGE ( 'NONE', *, *, #3699, .T. ) ;
#8571=CARTESIAN_POINT ( 'NONE',  ( -36.74999999999997158, 3.469446951953614189E-15, -6.938893903907228378E-15 ) ) ;
#8573=FACE_OUTER_BOUND ( 'NONE', #1038, .T. ) ;
#8593=CARTESIAN_POINT ( 'NONE',  ( -4.250000000000000888, 32.50000000000005684, -6.938893903907228378E-15 ) ) ;
#8595=DIRECTION ( 'NONE',  ( 3.851859888774471706E-33, -7.598173571352223877E-18, 1.000000000000000000 ) ) ;
#8601=DIRECTION ( 'NONE',  ( 1.000000000000000000, -1.284024588418159817E-35, 0.000000000000000000 ) ) ;
#8604=EDGE_CURVE ( 'NONE', #7000, #2630, #7703, .T. ) ;
#8643=COLOUR_RGB('Light Blue',0.38,0.62,0.78);
#8644=FILL_AREA_STYLE_COLOUR('',#8643);
#8645=FILL_AREA_STYLE('',(#8644));
#8646=SURFACE_STYLE_FILL_AREA(#8645);
#8647=SURFACE_SIDE_STYLE('',(#8646));
#8648=SURFACE_STYLE_USAGE(.BOTH.,#8647);
#8649=PRESENTATION_STYLE_ASSIGNMENT((#8648));
ENDSEC;
END-ISO-10303-21;
